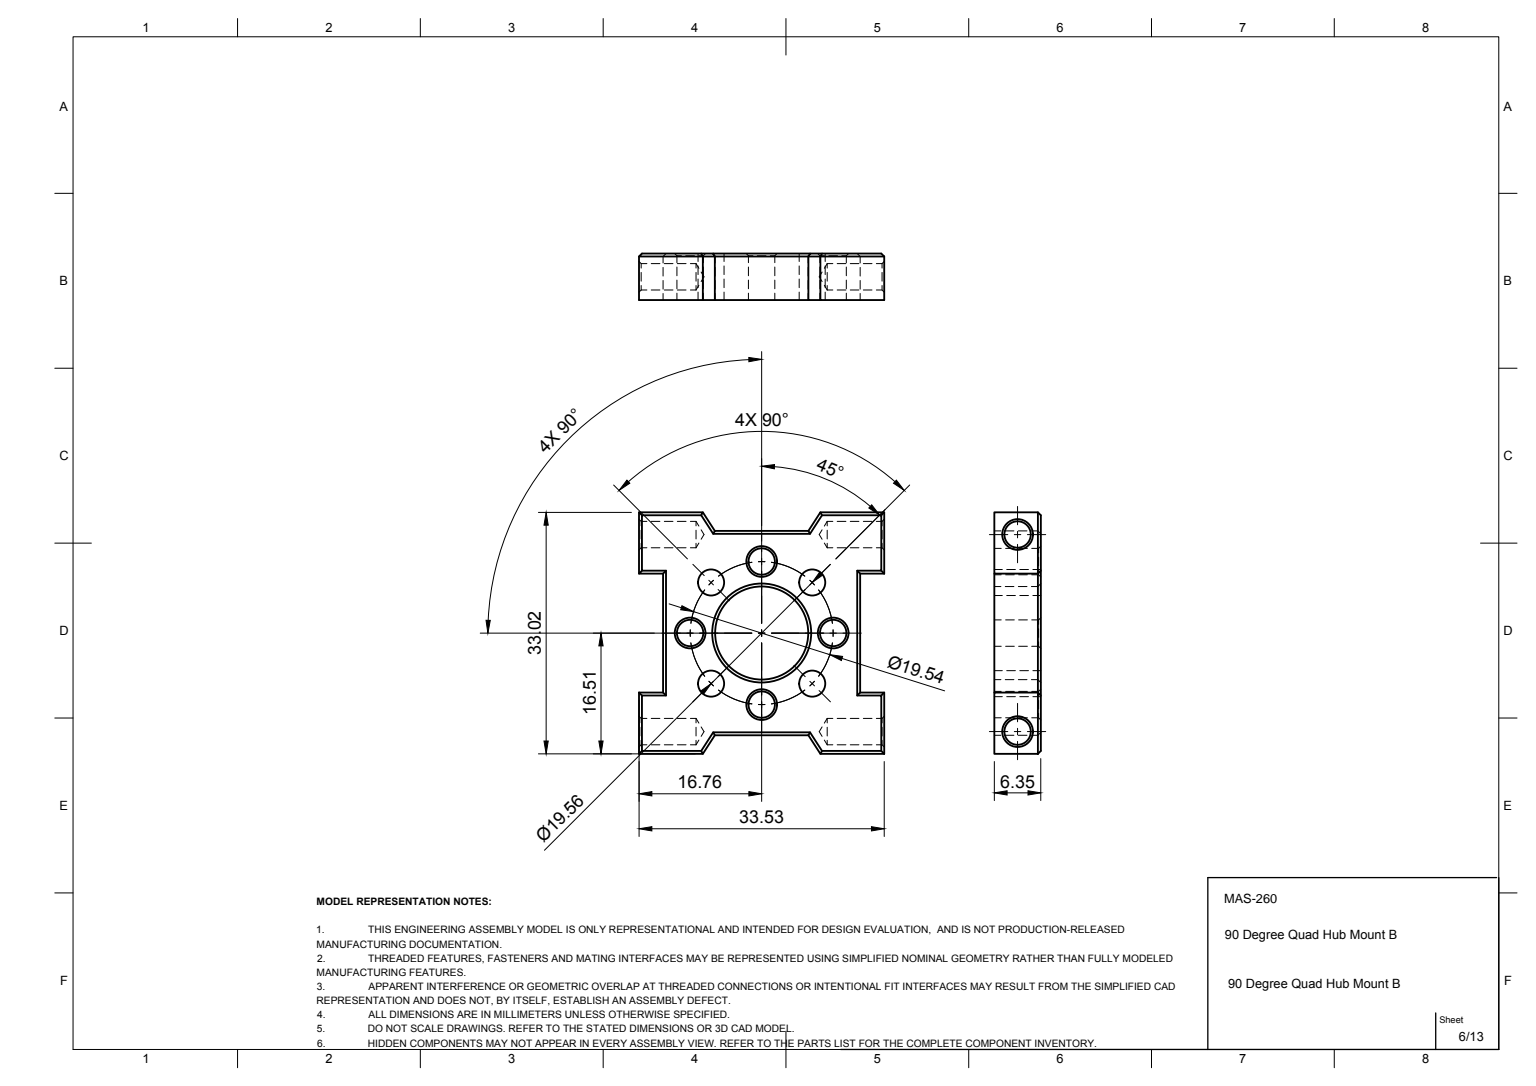
ISO-10303-21;
HEADER;
/* Generated by software containing ST-Developer
 * from STEP Tools, Inc. (www.steptools.com) 
 */

FILE_DESCRIPTION(
/* description */ (''),
/* implementation_level */ '2;1');

FILE_NAME(
/* name */ '90 Degree Quad Hub Mount B.step',
/* time_stamp */ '2026-10-15T13:29:10-07:00',
/* author */ (''),
/* organization */ (''),
/* preprocessor_version */ 'ST-DEVELOPER v20.2',
/* originating_system */ 'Autodesk Translation Framework v15.15.0.0',
/* authorisation */ '');

FILE_SCHEMA (('AUTOMOTIVE_DESIGN { 1 0 10303 214 3 1 1 }'));
ENDSEC;

DATA;
#10=MECHANICAL_DESIGN_GEOMETRIC_PRESENTATION_REPRESENTATION('',(#933),#83219);
#905=SHAPE_REPRESENTATION_RELATIONSHIP('SRR','None',#83300,#919);
#919=ADVANCED_BREP_SHAPE_REPRESENTATION('',(#947),#83205);
#933=STYLED_ITEM('',(#83379),#947);
#947=MANIFOLD_SOLID_BREP('Body1',#26929);
#961=FACE_BOUND('',#3739,.T.);
#962=FACE_BOUND('',#3743,.T.);
#963=FACE_BOUND('',#3749,.T.);
#964=FACE_BOUND('',#3753,.T.);
#965=FACE_BOUND('',#3762,.T.);
#966=FACE_BOUND('',#3763,.T.);
#967=FACE_BOUND('',#3764,.T.);
#968=FACE_BOUND('',#3765,.T.);
#969=FACE_BOUND('',#3766,.T.);
#970=FACE_BOUND('',#3767,.T.);
#971=FACE_BOUND('',#3768,.T.);
#972=FACE_BOUND('',#3769,.T.);
#973=FACE_BOUND('',#3770,.T.);
#974=FACE_BOUND('',#3814,.T.);
#975=FACE_BOUND('',#3815,.T.);
#976=FACE_BOUND('',#3816,.T.);
#977=FACE_BOUND('',#3817,.T.);
#978=FACE_BOUND('',#3818,.T.);
#979=FACE_BOUND('',#3819,.T.);
#980=FACE_BOUND('',#3820,.T.);
#981=FACE_BOUND('',#3821,.T.);
#982=FACE_BOUND('',#3822,.T.);
#1123=PLANE('',#27106);
#1124=PLANE('',#27113);
#1125=PLANE('',#27122);
#1126=PLANE('',#27129);
#1127=PLANE('',#27147);
#1128=PLANE('',#27170);
#1129=PLANE('',#27171);
#1130=PLANE('',#27172);
#1131=PLANE('',#27173);
#1132=PLANE('',#27174);
#1133=PLANE('',#27175);
#1134=PLANE('',#27176);
#1135=PLANE('',#27177);
#1136=PLANE('',#27178);
#1137=PLANE('',#27179);
#1138=PLANE('',#27180);
#1139=PLANE('',#27181);
#1140=PLANE('',#27182);
#1141=PLANE('',#27183);
#1142=PLANE('',#27184);
#1143=PLANE('',#27185);
#1144=PLANE('',#27186);
#1145=PLANE('',#27187);
#1146=PLANE('',#27188);
#1147=PLANE('',#27189);
#1148=PLANE('',#27190);
#1149=PLANE('',#27191);
#1150=PLANE('',#27192);
#1151=PLANE('',#27193);
#1152=PLANE('',#27194);
#1153=PLANE('',#27195);
#1154=PLANE('',#27196);
#1155=PLANE('',#27197);
#1156=PLANE('',#27198);
#1157=PLANE('',#27199);
#1158=PLANE('',#27200);
#1159=PLANE('',#27201);
#1160=PLANE('',#27202);
#1161=PLANE('',#27203);
#1162=PLANE('',#27204);
#1163=PLANE('',#27205);
#1164=PLANE('',#27206);
#2142=CYLINDRICAL_SURFACE('',#27103,1.8025);
#2143=CYLINDRICAL_SURFACE('',#27110,1.8025);
#2144=CYLINDRICAL_SURFACE('',#27119,1.8025);
#2145=CYLINDRICAL_SURFACE('',#27126,1.8025);
#2146=CYLINDRICAL_SURFACE('',#27132,1.778);
#2147=CYLINDRICAL_SURFACE('',#27135,1.778);
#2148=CYLINDRICAL_SURFACE('',#27138,1.778);
#2149=CYLINDRICAL_SURFACE('',#27141,1.778);
#2150=CYLINDRICAL_SURFACE('',#27152,1.8025);
#2151=CYLINDRICAL_SURFACE('',#27156,1.8025);
#2152=CYLINDRICAL_SURFACE('',#27160,1.8025);
#2153=CYLINDRICAL_SURFACE('',#27164,1.8025);
#2154=CYLINDRICAL_SURFACE('',#27168,6.363);
#2357=FACE_OUTER_BOUND('',#3736,.T.);
#2358=FACE_OUTER_BOUND('',#3737,.T.);
#2359=FACE_OUTER_BOUND('',#3738,.T.);
#2360=FACE_OUTER_BOUND('',#3740,.T.);
#2361=FACE_OUTER_BOUND('',#3741,.T.);
#2362=FACE_OUTER_BOUND('',#3742,.T.);
#2363=FACE_OUTER_BOUND('',#3744,.T.);
#2364=FACE_OUTER_BOUND('',#3745,.T.);
#2365=FACE_OUTER_BOUND('',#3746,.T.);
#2366=FACE_OUTER_BOUND('',#3747,.T.);
#2367=FACE_OUTER_BOUND('',#3748,.T.);
#2368=FACE_OUTER_BOUND('',#3750,.T.);
#2369=FACE_OUTER_BOUND('',#3751,.T.);
#2370=FACE_OUTER_BOUND('',#3752,.T.);
#2371=FACE_OUTER_BOUND('',#3754,.T.);
#2372=FACE_OUTER_BOUND('',#3755,.T.);
#2373=FACE_OUTER_BOUND('',#3756,.T.);
#2374=FACE_OUTER_BOUND('',#3757,.T.);
#2375=FACE_OUTER_BOUND('',#3758,.T.);
#2376=FACE_OUTER_BOUND('',#3759,.T.);
#2377=FACE_OUTER_BOUND('',#3760,.T.);
#2378=FACE_OUTER_BOUND('',#3761,.T.);
#2379=FACE_OUTER_BOUND('',#3771,.T.);
#2380=FACE_OUTER_BOUND('',#3772,.T.);
#2381=FACE_OUTER_BOUND('',#3773,.T.);
#2382=FACE_OUTER_BOUND('',#3774,.T.);
#2383=FACE_OUTER_BOUND('',#3775,.T.);
#2384=FACE_OUTER_BOUND('',#3776,.T.);
#2385=FACE_OUTER_BOUND('',#3777,.T.);
#2386=FACE_OUTER_BOUND('',#3778,.T.);
#2387=FACE_OUTER_BOUND('',#3779,.T.);
#2388=FACE_OUTER_BOUND('',#3780,.T.);
#2389=FACE_OUTER_BOUND('',#3781,.T.);
#2390=FACE_OUTER_BOUND('',#3782,.T.);
#2391=FACE_OUTER_BOUND('',#3783,.T.);
#2392=FACE_OUTER_BOUND('',#3784,.T.);
#2393=FACE_OUTER_BOUND('',#3785,.T.);
#2394=FACE_OUTER_BOUND('',#3786,.T.);
#2395=FACE_OUTER_BOUND('',#3787,.T.);
#2396=FACE_OUTER_BOUND('',#3788,.T.);
#2397=FACE_OUTER_BOUND('',#3789,.T.);
#2398=FACE_OUTER_BOUND('',#3790,.T.);
#2399=FACE_OUTER_BOUND('',#3791,.T.);
#2400=FACE_OUTER_BOUND('',#3792,.T.);
#2401=FACE_OUTER_BOUND('',#3793,.T.);
#2402=FACE_OUTER_BOUND('',#3794,.T.);
#2403=FACE_OUTER_BOUND('',#3795,.T.);
#2404=FACE_OUTER_BOUND('',#3796,.T.);
#2405=FACE_OUTER_BOUND('',#3797,.T.);
#2406=FACE_OUTER_BOUND('',#3798,.T.);
#2407=FACE_OUTER_BOUND('',#3799,.T.);
#2408=FACE_OUTER_BOUND('',#3800,.T.);
#2409=FACE_OUTER_BOUND('',#3801,.T.);
#2410=FACE_OUTER_BOUND('',#3802,.T.);
#2411=FACE_OUTER_BOUND('',#3803,.T.);
#2412=FACE_OUTER_BOUND('',#3804,.T.);
#2413=FACE_OUTER_BOUND('',#3805,.T.);
#2414=FACE_OUTER_BOUND('',#3806,.T.);
#2415=FACE_OUTER_BOUND('',#3807,.T.);
#2416=FACE_OUTER_BOUND('',#3808,.T.);
#2417=FACE_OUTER_BOUND('',#3809,.T.);
#2418=FACE_OUTER_BOUND('',#3810,.T.);
#2419=FACE_OUTER_BOUND('',#3811,.T.);
#2420=FACE_OUTER_BOUND('',#3812,.T.);
#2421=FACE_OUTER_BOUND('',#3813,.T.);
#2422=FACE_OUTER_BOUND('',#3823,.T.);
#2423=FACE_OUTER_BOUND('',#3824,.T.);
#2424=FACE_OUTER_BOUND('',#3825,.T.);
#3736=EDGE_LOOP('',(#17586,#17587,#17588,#17589));
#3737=EDGE_LOOP('',(#17590,#17591,#17592,#17593,#17594));
#3738=EDGE_LOOP('',(#17595,#17596,#17597,#17598));
#3739=EDGE_LOOP('',(#17599));
#3740=EDGE_LOOP('',(#17600,#17601,#17602,#17603));
#3741=EDGE_LOOP('',(#17604,#17605,#17606,#17607,#17608));
#3742=EDGE_LOOP('',(#17609,#17610,#17611,#17612));
#3743=EDGE_LOOP('',(#17613));
#3744=EDGE_LOOP('',(#17614,#17615,#17616,#17617));
#3745=EDGE_LOOP('',(#17618,#17619,#17620,#17621));
#3746=EDGE_LOOP('',(#17622,#17623,#17624,#17625));
#3747=EDGE_LOOP('',(#17626,#17627,#17628,#17629,#17630));
#3748=EDGE_LOOP('',(#17631,#17632,#17633,#17634));
#3749=EDGE_LOOP('',(#17635));
#3750=EDGE_LOOP('',(#17636,#17637,#17638,#17639));
#3751=EDGE_LOOP('',(#17640,#17641,#17642,#17643,#17644));
#3752=EDGE_LOOP('',(#17645,#17646,#17647,#17648));
#3753=EDGE_LOOP('',(#17649));
#3754=EDGE_LOOP('',(#17650,#17651,#17652,#17653));
#3755=EDGE_LOOP('',(#17654,#17655,#17656,#17657));
#3756=EDGE_LOOP('',(#17658,#17659,#17660,#17661));
#3757=EDGE_LOOP('',(#17662,#17663,#17664,#17665));
#3758=EDGE_LOOP('',(#17666,#17667,#17668,#17669));
#3759=EDGE_LOOP('',(#17670,#17671,#17672,#17673));
#3760=EDGE_LOOP('',(#17674,#17675,#17676,#17677));
#3761=EDGE_LOOP('',(#17678,#17679,#17680,#17681,#17682,#17683,#17684,#17685,
#17686,#17687,#17688,#17689,#17690,#17691,#17692,#17693,#17694,#17695,#17696,
#17697));
#3762=EDGE_LOOP('',(#17698));
#3763=EDGE_LOOP('',(#17699));
#3764=EDGE_LOOP('',(#17700));
#3765=EDGE_LOOP('',(#17701));
#3766=EDGE_LOOP('',(#17702));
#3767=EDGE_LOOP('',(#17703));
#3768=EDGE_LOOP('',(#17704));
#3769=EDGE_LOOP('',(#17705));
#3770=EDGE_LOOP('',(#17706));
#3771=EDGE_LOOP('',(#17707,#17708,#17709,#17710));
#3772=EDGE_LOOP('',(#17711,#17712,#17713,#17714));
#3773=EDGE_LOOP('',(#17715,#17716,#17717,#17718));
#3774=EDGE_LOOP('',(#17719,#17720,#17721,#17722));
#3775=EDGE_LOOP('',(#17723,#17724,#17725,#17726));
#3776=EDGE_LOOP('',(#17727,#17728,#17729,#17730));
#3777=EDGE_LOOP('',(#17731,#17732,#17733,#17734));
#3778=EDGE_LOOP('',(#17735,#17736,#17737,#17738));
#3779=EDGE_LOOP('',(#17739,#17740,#17741,#17742));
#3780=EDGE_LOOP('',(#17743,#17744,#17745,#17746));
#3781=EDGE_LOOP('',(#17747,#17748,#17749,#17750));
#3782=EDGE_LOOP('',(#17751,#17752,#17753,#17754));
#3783=EDGE_LOOP('',(#17755,#17756,#17757,#17758));
#3784=EDGE_LOOP('',(#17759,#17760,#17761,#17762));
#3785=EDGE_LOOP('',(#17763,#17764,#17765,#17766));
#3786=EDGE_LOOP('',(#17767,#17768,#17769,#17770));
#3787=EDGE_LOOP('',(#17771,#17772,#17773,#17774));
#3788=EDGE_LOOP('',(#17775,#17776,#17777,#17778));
#3789=EDGE_LOOP('',(#17779,#17780,#17781,#17782));
#3790=EDGE_LOOP('',(#17783,#17784,#17785,#17786));
#3791=EDGE_LOOP('',(#17787,#17788,#17789,#17790));
#3792=EDGE_LOOP('',(#17791,#17792,#17793,#17794));
#3793=EDGE_LOOP('',(#17795,#17796,#17797,#17798));
#3794=EDGE_LOOP('',(#17799,#17800,#17801,#17802));
#3795=EDGE_LOOP('',(#17803,#17804,#17805,#17806));
#3796=EDGE_LOOP('',(#17807,#17808,#17809,#17810));
#3797=EDGE_LOOP('',(#17811,#17812,#17813,#17814));
#3798=EDGE_LOOP('',(#17815,#17816,#17817,#17818));
#3799=EDGE_LOOP('',(#17819,#17820,#17821,#17822));
#3800=EDGE_LOOP('',(#17823,#17824,#17825,#17826));
#3801=EDGE_LOOP('',(#17827,#17828,#17829,#17830));
#3802=EDGE_LOOP('',(#17831,#17832,#17833,#17834));
#3803=EDGE_LOOP('',(#17835,#17836,#17837,#17838));
#3804=EDGE_LOOP('',(#17839,#17840,#17841,#17842));
#3805=EDGE_LOOP('',(#17843,#17844,#17845,#17846));
#3806=EDGE_LOOP('',(#17847,#17848,#17849,#17850));
#3807=EDGE_LOOP('',(#17851,#17852,#17853,#17854));
#3808=EDGE_LOOP('',(#17855,#17856,#17857,#17858));
#3809=EDGE_LOOP('',(#17859,#17860,#17861,#17862));
#3810=EDGE_LOOP('',(#17863,#17864,#17865,#17866));
#3811=EDGE_LOOP('',(#17867,#17868,#17869,#17870));
#3812=EDGE_LOOP('',(#17871,#17872,#17873,#17874));
#3813=EDGE_LOOP('',(#17875,#17876,#17877,#17878,#17879,#17880,#17881,#17882,
#17883,#17884,#17885,#17886,#17887,#17888,#17889,#17890,#17891,#17892,#17893,
#17894));
#3814=EDGE_LOOP('',(#17895));
#3815=EDGE_LOOP('',(#17896));
#3816=EDGE_LOOP('',(#17897));
#3817=EDGE_LOOP('',(#17898));
#3818=EDGE_LOOP('',(#17899));
#3819=EDGE_LOOP('',(#17900));
#3820=EDGE_LOOP('',(#17901));
#3821=EDGE_LOOP('',(#17902));
#3822=EDGE_LOOP('',(#17903));
#3823=EDGE_LOOP('',(#17904,#17905,#17906,#17907));
#3824=EDGE_LOOP('',(#17908,#17909,#17910,#17911));
#3825=EDGE_LOOP('',(#17912,#17913,#17914,#17915));
#5277=LINE('',#36086,#7788);
#5278=LINE('',#36090,#7789);
#5279=LINE('',#36097,#7790);
#5280=LINE('',#36099,#7791);
#5281=LINE('',#36101,#7792);
#5282=LINE('',#36102,#7793);
#5283=LINE('',#36107,#7794);
#5284=LINE('',#36111,#7795);
#5285=LINE('',#36118,#7796);
#5286=LINE('',#36120,#7797);
#5287=LINE('',#36122,#7798);
#5288=LINE('',#36123,#7799);
#5289=LINE('',#36126,#7800);
#5290=LINE('',#36129,#7801);
#5291=LINE('',#36134,#7802);
#5292=LINE('',#36138,#7803);
#5293=LINE('',#36145,#7804);
#5294=LINE('',#36147,#7805);
#5295=LINE('',#36149,#7806);
#5296=LINE('',#36150,#7807);
#5297=LINE('',#36155,#7808);
#5298=LINE('',#36159,#7809);
#5299=LINE('',#36166,#7810);
#5300=LINE('',#36168,#7811);
#5301=LINE('',#36170,#7812);
#5302=LINE('',#36171,#7813);
#5303=LINE('',#36174,#7814);
#5304=LINE('',#36177,#7815);
#5305=LINE('',#36182,#7816);
#5306=LINE('',#36188,#7817);
#5307=LINE('',#36194,#7818);
#5308=LINE('',#36200,#7819);
#5309=LINE('',#36206,#7820);
#5310=LINE('',#36211,#7821);
#5311=LINE('',#36213,#7822);
#5312=LINE('',#36215,#7823);
#5313=LINE('',#36217,#7824);
#5314=LINE('',#36219,#7825);
#5315=LINE('',#36221,#7826);
#5316=LINE('',#36223,#7827);
#5317=LINE('',#36225,#7828);
#5318=LINE('',#36227,#7829);
#5319=LINE('',#36229,#7830);
#5320=LINE('',#36231,#7831);
#5321=LINE('',#36233,#7832);
#5322=LINE('',#36235,#7833);
#5323=LINE('',#36237,#7834);
#5324=LINE('',#36239,#7835);
#5325=LINE('',#36241,#7836);
#5326=LINE('',#36243,#7837);
#5327=LINE('',#36245,#7838);
#5328=LINE('',#36247,#7839);
#5329=LINE('',#36248,#7840);
#5330=LINE('',#36259,#7841);
#5331=LINE('',#36264,#7842);
#5332=LINE('',#36267,#7843);
#5333=LINE('',#36272,#7844);
#5334=LINE('',#36275,#7845);
#5335=LINE('',#36280,#7846);
#5336=LINE('',#36283,#7847);
#5337=LINE('',#36288,#7848);
#5338=LINE('',#36291,#7849);
#5339=LINE('',#36295,#7850);
#5340=LINE('',#36297,#7851);
#5341=LINE('',#36298,#7852);
#5342=LINE('',#36300,#7853);
#5343=LINE('',#36301,#7854);
#5344=LINE('',#36303,#7855);
#5345=LINE('',#36307,#7856);
#5346=LINE('',#36308,#7857);
#5347=LINE('',#36309,#7858);
#5348=LINE('',#36312,#7859);
#5349=LINE('',#36313,#7860);
#5350=LINE('',#36315,#7861);
#5351=LINE('',#36317,#7862);
#5352=LINE('',#36318,#7863);
#5353=LINE('',#36320,#7864);
#5354=LINE('',#36324,#7865);
#5355=LINE('',#36325,#7866);
#5356=LINE('',#36326,#7867);
#5357=LINE('',#36329,#7868);
#5358=LINE('',#36330,#7869);
#5359=LINE('',#36333,#7870);
#5360=LINE('',#36334,#7871);
#5361=LINE('',#36336,#7872);
#5362=LINE('',#36338,#7873);
#5363=LINE('',#36339,#7874);
#5364=LINE('',#36341,#7875);
#5365=LINE('',#36343,#7876);
#5366=LINE('',#36345,#7877);
#5367=LINE('',#36347,#7878);
#5368=LINE('',#36348,#7879);
#5369=LINE('',#36350,#7880);
#5370=LINE('',#36353,#7881);
#5371=LINE('',#36354,#7882);
#5372=LINE('',#36357,#7883);
#5373=LINE('',#36358,#7884);
#5374=LINE('',#36360,#7885);
#5375=LINE('',#36363,#7886);
#5376=LINE('',#36364,#7887);
#5377=LINE('',#36367,#7888);
#5378=LINE('',#36368,#7889);
#5379=LINE('',#36371,#7890);
#5380=LINE('',#36372,#7891);
#5381=LINE('',#36374,#7892);
#5382=LINE('',#36377,#7893);
#5383=LINE('',#36378,#7894);
#5384=LINE('',#36381,#7895);
#5385=LINE('',#36382,#7896);
#5386=LINE('',#36385,#7897);
#5387=LINE('',#36386,#7898);
#5388=LINE('',#36389,#7899);
#5389=LINE('',#36390,#7900);
#5390=LINE('',#36393,#7901);
#5391=LINE('',#36395,#7902);
#5392=LINE('',#36396,#7903);
#5393=LINE('',#36399,#7904);
#5394=LINE('',#36400,#7905);
#5395=LINE('',#36402,#7906);
#5396=LINE('',#36404,#7907);
#5397=LINE('',#36406,#7908);
#5398=LINE('',#36409,#7909);
#5399=LINE('',#36411,#7910);
#5400=LINE('',#36412,#7911);
#5401=LINE('',#36414,#7912);
#5402=LINE('',#36415,#7913);
#7788=VECTOR('',#29263,1.9525);
#7789=VECTOR('',#29268,1.8025);
#7790=VECTOR('',#29275,10.);
#7791=VECTOR('',#29276,10.);
#7792=VECTOR('',#29277,10.);
#7793=VECTOR('',#29278,10.);
#7794=VECTOR('',#29283,1.9525);
#7795=VECTOR('',#29288,1.8025);
#7796=VECTOR('',#29295,10.);
#7797=VECTOR('',#29296,10.);
#7798=VECTOR('',#29297,10.);
#7799=VECTOR('',#29298,10.);
#7800=VECTOR('',#29301,1.80249999999999);
#7801=VECTOR('',#29304,1.80249999999999);
#7802=VECTOR('',#29309,1.9525);
#7803=VECTOR('',#29314,1.8025);
#7804=VECTOR('',#29321,10.);
#7805=VECTOR('',#29322,10.);
#7806=VECTOR('',#29323,10.);
#7807=VECTOR('',#29324,10.);
#7808=VECTOR('',#29329,1.9525);
#7809=VECTOR('',#29334,1.8025);
#7810=VECTOR('',#29341,10.);
#7811=VECTOR('',#29342,10.);
#7812=VECTOR('',#29343,10.);
#7813=VECTOR('',#29344,10.);
#7814=VECTOR('',#29347,0.901249999999996);
#7815=VECTOR('',#29350,0.901249999999996);
#7816=VECTOR('',#29355,1.778);
#7817=VECTOR('',#29362,1.778);
#7818=VECTOR('',#29369,1.778);
#7819=VECTOR('',#29376,1.778);
#7820=VECTOR('',#29383,1.9525);
#7821=VECTOR('',#29388,10.);
#7822=VECTOR('',#29389,10.);
#7823=VECTOR('',#29390,10.);
#7824=VECTOR('',#29391,10.);
#7825=VECTOR('',#29392,10.);
#7826=VECTOR('',#29393,10.);
#7827=VECTOR('',#29394,10.);
#7828=VECTOR('',#29395,10.);
#7829=VECTOR('',#29396,10.);
#7830=VECTOR('',#29397,10.);
#7831=VECTOR('',#29398,10.);
#7832=VECTOR('',#29399,10.);
#7833=VECTOR('',#29400,10.);
#7834=VECTOR('',#29401,10.);
#7835=VECTOR('',#29402,10.);
#7836=VECTOR('',#29403,10.);
#7837=VECTOR('',#29404,10.);
#7838=VECTOR('',#29405,10.);
#7839=VECTOR('',#29406,10.);
#7840=VECTOR('',#29407,10.);
#7841=VECTOR('',#29418,1.8025);
#7842=VECTOR('',#29425,1.9525);
#7843=VECTOR('',#29428,1.8025);
#7844=VECTOR('',#29435,1.9525);
#7845=VECTOR('',#29438,1.8025);
#7846=VECTOR('',#29445,1.9525);
#7847=VECTOR('',#29448,1.8025);
#7848=VECTOR('',#29455,6.563);
#7849=VECTOR('',#29458,6.363);
#7850=VECTOR('',#29463,10.);
#7851=VECTOR('',#29464,10.);
#7852=VECTOR('',#29465,10.);
#7853=VECTOR('',#29468,9.99999999999999);
#7854=VECTOR('',#29469,10.);
#7855=VECTOR('',#29472,10.);
#7856=VECTOR('',#29475,10.);
#7857=VECTOR('',#29476,10.);
#7858=VECTOR('',#29477,10.);
#7859=VECTOR('',#29480,10.);
#7860=VECTOR('',#29481,10.);
#7861=VECTOR('',#29484,10.);
#7862=VECTOR('',#29485,10.);
#7863=VECTOR('',#29486,10.);
#7864=VECTOR('',#29489,10.);
#7865=VECTOR('',#29492,10.);
#7866=VECTOR('',#29493,10.);
#7867=VECTOR('',#29494,10.);
#7868=VECTOR('',#29497,10.);
#7869=VECTOR('',#29498,10.);
#7870=VECTOR('',#29501,10.);
#7871=VECTOR('',#29502,10.);
#7872=VECTOR('',#29505,10.);
#7873=VECTOR('',#29508,10.);
#7874=VECTOR('',#29509,9.99999999999999);
#7875=VECTOR('',#29512,10.);
#7876=VECTOR('',#29515,10.);
#7877=VECTOR('',#29518,10.);
#7878=VECTOR('',#29521,10.);
#7879=VECTOR('',#29522,10.);
#7880=VECTOR('',#29525,10.);
#7881=VECTOR('',#29528,10.);
#7882=VECTOR('',#29529,10.);
#7883=VECTOR('',#29532,10.);
#7884=VECTOR('',#29533,10.);
#7885=VECTOR('',#29536,10.);
#7886=VECTOR('',#29539,10.);
#7887=VECTOR('',#29540,10.);
#7888=VECTOR('',#29543,10.);
#7889=VECTOR('',#29544,10.);
#7890=VECTOR('',#29547,10.);
#7891=VECTOR('',#29548,10.);
#7892=VECTOR('',#29551,10.);
#7893=VECTOR('',#29554,10.);
#7894=VECTOR('',#29555,10.);
#7895=VECTOR('',#29558,10.);
#7896=VECTOR('',#29559,10.);
#7897=VECTOR('',#29562,10.);
#7898=VECTOR('',#29563,10.);
#7899=VECTOR('',#29566,10.);
#7900=VECTOR('',#29567,10.);
#7901=VECTOR('',#29570,10.);
#7902=VECTOR('',#29571,10.);
#7903=VECTOR('',#29572,10.);
#7904=VECTOR('',#29575,10.);
#7905=VECTOR('',#29576,10.);
#7906=VECTOR('',#29579,10.);
#7907=VECTOR('',#29582,10.);
#7908=VECTOR('',#29585,10.);
#7909=VECTOR('',#29588,10.);
#7910=VECTOR('',#29589,10.);
#7911=VECTOR('',#29590,10.);
#7912=VECTOR('',#29593,10.);
#7913=VECTOR('',#29594,10.);
#10299=CIRCLE('',#27101,1.8025);
#10300=CIRCLE('',#27102,2.1025);
#10301=CIRCLE('',#27104,1.8025);
#10302=CIRCLE('',#27105,1.8025);
#10303=CIRCLE('',#27108,1.8025);
#10304=CIRCLE('',#27109,2.1025);
#10305=CIRCLE('',#27111,1.8025);
#10306=CIRCLE('',#27112,1.8025);
#10307=CIRCLE('',#27117,1.8025);
#10308=CIRCLE('',#27118,2.1025);
#10309=CIRCLE('',#27120,1.8025);
#10310=CIRCLE('',#27121,1.8025);
#10311=CIRCLE('',#27124,1.8025);
#10312=CIRCLE('',#27125,2.1025);
#10313=CIRCLE('',#27127,1.8025);
#10314=CIRCLE('',#27128,1.8025);
#10315=CIRCLE('',#27133,1.778);
#10316=CIRCLE('',#27134,1.778);
#10317=CIRCLE('',#27136,1.778);
#10318=CIRCLE('',#27137,1.778);
#10319=CIRCLE('',#27139,1.778);
#10320=CIRCLE('',#27140,1.778);
#10321=CIRCLE('',#27142,1.778);
#10322=CIRCLE('',#27143,1.778);
#10323=CIRCLE('',#27145,1.8025);
#10324=CIRCLE('',#27146,2.1025);
#10325=CIRCLE('',#27148,2.1025);
#10326=CIRCLE('',#27149,6.763);
#10327=CIRCLE('',#27150,2.1025);
#10328=CIRCLE('',#27151,2.1025);
#10329=CIRCLE('',#27153,1.8025);
#10330=CIRCLE('',#27155,1.8025);
#10331=CIRCLE('',#27157,1.8025);
#10332=CIRCLE('',#27159,1.8025);
#10333=CIRCLE('',#27161,1.8025);
#10334=CIRCLE('',#27163,1.8025);
#10335=CIRCLE('',#27165,1.8025);
#10336=CIRCLE('',#27167,6.363);
#10337=CIRCLE('',#27169,6.363);
#11051=VERTEX_POINT('',#36083);
#11052=VERTEX_POINT('',#36085);
#11053=VERTEX_POINT('',#36089);
#11054=VERTEX_POINT('',#36091);
#11055=VERTEX_POINT('',#36095);
#11056=VERTEX_POINT('',#36096);
#11057=VERTEX_POINT('',#36098);
#11058=VERTEX_POINT('',#36100);
#11059=VERTEX_POINT('',#36104);
#11060=VERTEX_POINT('',#36106);
#11061=VERTEX_POINT('',#36110);
#11062=VERTEX_POINT('',#36112);
#11063=VERTEX_POINT('',#36116);
#11064=VERTEX_POINT('',#36117);
#11065=VERTEX_POINT('',#36119);
#11066=VERTEX_POINT('',#36121);
#11067=VERTEX_POINT('',#36125);
#11068=VERTEX_POINT('',#36128);
#11069=VERTEX_POINT('',#36131);
#11070=VERTEX_POINT('',#36133);
#11071=VERTEX_POINT('',#36137);
#11072=VERTEX_POINT('',#36139);
#11073=VERTEX_POINT('',#36143);
#11074=VERTEX_POINT('',#36144);
#11075=VERTEX_POINT('',#36146);
#11076=VERTEX_POINT('',#36148);
#11077=VERTEX_POINT('',#36152);
#11078=VERTEX_POINT('',#36154);
#11079=VERTEX_POINT('',#36158);
#11080=VERTEX_POINT('',#36160);
#11081=VERTEX_POINT('',#36164);
#11082=VERTEX_POINT('',#36165);
#11083=VERTEX_POINT('',#36167);
#11084=VERTEX_POINT('',#36169);
#11085=VERTEX_POINT('',#36173);
#11086=VERTEX_POINT('',#36176);
#11087=VERTEX_POINT('',#36179);
#11088=VERTEX_POINT('',#36181);
#11089=VERTEX_POINT('',#36185);
#11090=VERTEX_POINT('',#36187);
#11091=VERTEX_POINT('',#36191);
#11092=VERTEX_POINT('',#36193);
#11093=VERTEX_POINT('',#36197);
#11094=VERTEX_POINT('',#36199);
#11095=VERTEX_POINT('',#36203);
#11096=VERTEX_POINT('',#36205);
#11097=VERTEX_POINT('',#36209);
#11098=VERTEX_POINT('',#36210);
#11099=VERTEX_POINT('',#36212);
#11100=VERTEX_POINT('',#36214);
#11101=VERTEX_POINT('',#36216);
#11102=VERTEX_POINT('',#36218);
#11103=VERTEX_POINT('',#36220);
#11104=VERTEX_POINT('',#36222);
#11105=VERTEX_POINT('',#36224);
#11106=VERTEX_POINT('',#36226);
#11107=VERTEX_POINT('',#36228);
#11108=VERTEX_POINT('',#36230);
#11109=VERTEX_POINT('',#36232);
#11110=VERTEX_POINT('',#36234);
#11111=VERTEX_POINT('',#36236);
#11112=VERTEX_POINT('',#36238);
#11113=VERTEX_POINT('',#36240);
#11114=VERTEX_POINT('',#36242);
#11115=VERTEX_POINT('',#36244);
#11116=VERTEX_POINT('',#36246);
#11117=VERTEX_POINT('',#36249);
#11118=VERTEX_POINT('',#36251);
#11119=VERTEX_POINT('',#36253);
#11120=VERTEX_POINT('',#36255);
#11121=VERTEX_POINT('',#36258);
#11122=VERTEX_POINT('',#36262);
#11123=VERTEX_POINT('',#36266);
#11124=VERTEX_POINT('',#36270);
#11125=VERTEX_POINT('',#36274);
#11126=VERTEX_POINT('',#36278);
#11127=VERTEX_POINT('',#36282);
#11128=VERTEX_POINT('',#36286);
#11129=VERTEX_POINT('',#36290);
#11130=VERTEX_POINT('',#36294);
#11131=VERTEX_POINT('',#36296);
#11132=VERTEX_POINT('',#36305);
#11133=VERTEX_POINT('',#36306);
#11134=VERTEX_POINT('',#36311);
#11135=VERTEX_POINT('',#36316);
#11136=VERTEX_POINT('',#36322);
#11137=VERTEX_POINT('',#36323);
#11138=VERTEX_POINT('',#36328);
#11139=VERTEX_POINT('',#36332);
#11140=VERTEX_POINT('',#36352);
#11141=VERTEX_POINT('',#36356);
#11142=VERTEX_POINT('',#36362);
#11143=VERTEX_POINT('',#36366);
#11144=VERTEX_POINT('',#36370);
#11145=VERTEX_POINT('',#36376);
#11146=VERTEX_POINT('',#36380);
#11147=VERTEX_POINT('',#36384);
#11148=VERTEX_POINT('',#36388);
#11149=VERTEX_POINT('',#36392);
#11150=VERTEX_POINT('',#36394);
#11151=VERTEX_POINT('',#36398);
#11152=VERTEX_POINT('',#36408);
#11153=VERTEX_POINT('',#36410);
#13654=EDGE_CURVE('',#11051,#11051,#10299,.T.);
#13655=EDGE_CURVE('',#11051,#11052,#5277,.T.);
#13656=EDGE_CURVE('',#11052,#11052,#10300,.T.);
#13657=EDGE_CURVE('',#11051,#11053,#5278,.T.);
#13658=EDGE_CURVE('',#11053,#11054,#10301,.T.);
#13659=EDGE_CURVE('',#11054,#11053,#10302,.T.);
#13660=EDGE_CURVE('',#11055,#11056,#5279,.T.);
#13661=EDGE_CURVE('',#11057,#11055,#5280,.T.);
#13662=EDGE_CURVE('',#11058,#11057,#5281,.T.);
#13663=EDGE_CURVE('',#11058,#11056,#5282,.T.);
#13664=EDGE_CURVE('',#11059,#11059,#10303,.T.);
#13665=EDGE_CURVE('',#11059,#11060,#5283,.T.);
#13666=EDGE_CURVE('',#11060,#11060,#10304,.T.);
#13667=EDGE_CURVE('',#11059,#11061,#5284,.T.);
#13668=EDGE_CURVE('',#11061,#11062,#10305,.T.);
#13669=EDGE_CURVE('',#11062,#11061,#10306,.T.);
#13670=EDGE_CURVE('',#11063,#11064,#5285,.T.);
#13671=EDGE_CURVE('',#11063,#11065,#5286,.T.);
#13672=EDGE_CURVE('',#11066,#11065,#5287,.T.);
#13673=EDGE_CURVE('',#11066,#11064,#5288,.T.);
#13674=EDGE_CURVE('',#11067,#11054,#5289,.T.);
#13675=EDGE_CURVE('',#11068,#11062,#5290,.T.);
#13676=EDGE_CURVE('',#11069,#11069,#10307,.T.);
#13677=EDGE_CURVE('',#11069,#11070,#5291,.T.);
#13678=EDGE_CURVE('',#11070,#11070,#10308,.T.);
#13679=EDGE_CURVE('',#11069,#11071,#5292,.T.);
#13680=EDGE_CURVE('',#11071,#11072,#10309,.T.);
#13681=EDGE_CURVE('',#11072,#11071,#10310,.T.);
#13682=EDGE_CURVE('',#11073,#11074,#5293,.T.);
#13683=EDGE_CURVE('',#11073,#11075,#5294,.T.);
#13684=EDGE_CURVE('',#11076,#11075,#5295,.T.);
#13685=EDGE_CURVE('',#11076,#11074,#5296,.T.);
#13686=EDGE_CURVE('',#11077,#11077,#10311,.T.);
#13687=EDGE_CURVE('',#11077,#11078,#5297,.T.);
#13688=EDGE_CURVE('',#11078,#11078,#10312,.T.);
#13689=EDGE_CURVE('',#11077,#11079,#5298,.T.);
#13690=EDGE_CURVE('',#11079,#11080,#10313,.T.);
#13691=EDGE_CURVE('',#11080,#11079,#10314,.T.);
#13692=EDGE_CURVE('',#11081,#11082,#5299,.T.);
#13693=EDGE_CURVE('',#11083,#11081,#5300,.T.);
#13694=EDGE_CURVE('',#11084,#11083,#5301,.T.);
#13695=EDGE_CURVE('',#11084,#11082,#5302,.T.);
#13696=EDGE_CURVE('',#11085,#11072,#5303,.T.);
#13697=EDGE_CURVE('',#11086,#11080,#5304,.T.);
#13698=EDGE_CURVE('',#11087,#11087,#10315,.T.);
#13699=EDGE_CURVE('',#11087,#11088,#5305,.T.);
#13700=EDGE_CURVE('',#11088,#11088,#10316,.T.);
#13701=EDGE_CURVE('',#11089,#11089,#10317,.T.);
#13702=EDGE_CURVE('',#11089,#11090,#5306,.T.);
#13703=EDGE_CURVE('',#11090,#11090,#10318,.T.);
#13704=EDGE_CURVE('',#11091,#11091,#10319,.T.);
#13705=EDGE_CURVE('',#11091,#11092,#5307,.T.);
#13706=EDGE_CURVE('',#11092,#11092,#10320,.T.);
#13707=EDGE_CURVE('',#11093,#11093,#10321,.T.);
#13708=EDGE_CURVE('',#11093,#11094,#5308,.T.);
#13709=EDGE_CURVE('',#11094,#11094,#10322,.T.);
#13710=EDGE_CURVE('',#11095,#11095,#10323,.T.);
#13711=EDGE_CURVE('',#11095,#11096,#5309,.T.);
#13712=EDGE_CURVE('',#11096,#11096,#10324,.T.);
#13713=EDGE_CURVE('',#11097,#11098,#5310,.T.);
#13714=EDGE_CURVE('',#11099,#11097,#5311,.T.);
#13715=EDGE_CURVE('',#11100,#11099,#5312,.T.);
#13716=EDGE_CURVE('',#11101,#11100,#5313,.T.);
#13717=EDGE_CURVE('',#11102,#11101,#5314,.T.);
#13718=EDGE_CURVE('',#11103,#11102,#5315,.T.);
#13719=EDGE_CURVE('',#11104,#11103,#5316,.T.);
#13720=EDGE_CURVE('',#11105,#11104,#5317,.T.);
#13721=EDGE_CURVE('',#11106,#11105,#5318,.T.);
#13722=EDGE_CURVE('',#11107,#11106,#5319,.T.);
#13723=EDGE_CURVE('',#11108,#11107,#5320,.T.);
#13724=EDGE_CURVE('',#11109,#11108,#5321,.T.);
#13725=EDGE_CURVE('',#11110,#11109,#5322,.T.);
#13726=EDGE_CURVE('',#11111,#11110,#5323,.T.);
#13727=EDGE_CURVE('',#11112,#11111,#5324,.T.);
#13728=EDGE_CURVE('',#11113,#11112,#5325,.T.);
#13729=EDGE_CURVE('',#11114,#11113,#5326,.T.);
#13730=EDGE_CURVE('',#11115,#11114,#5327,.T.);
#13731=EDGE_CURVE('',#11116,#11115,#5328,.T.);
#13732=EDGE_CURVE('',#11098,#11116,#5329,.T.);
#13733=EDGE_CURVE('',#11117,#11117,#10325,.T.);
#13734=EDGE_CURVE('',#11118,#11118,#10326,.T.);
#13735=EDGE_CURVE('',#11119,#11119,#10327,.T.);
#13736=EDGE_CURVE('',#11120,#11120,#10328,.T.);
#13737=EDGE_CURVE('',#11095,#11121,#5330,.T.);
#13738=EDGE_CURVE('',#11121,#11121,#10329,.T.);
#13739=EDGE_CURVE('',#11122,#11122,#10330,.T.);
#13740=EDGE_CURVE('',#11122,#11120,#5331,.T.);
#13741=EDGE_CURVE('',#11122,#11123,#5332,.T.);
#13742=EDGE_CURVE('',#11123,#11123,#10331,.T.);
#13743=EDGE_CURVE('',#11124,#11124,#10332,.T.);
#13744=EDGE_CURVE('',#11124,#11117,#5333,.T.);
#13745=EDGE_CURVE('',#11124,#11125,#5334,.T.);
#13746=EDGE_CURVE('',#11125,#11125,#10333,.T.);
#13747=EDGE_CURVE('',#11126,#11126,#10334,.T.);
#13748=EDGE_CURVE('',#11126,#11119,#5335,.T.);
#13749=EDGE_CURVE('',#11126,#11127,#5336,.T.);
#13750=EDGE_CURVE('',#11127,#11127,#10335,.T.);
#13751=EDGE_CURVE('',#11128,#11128,#10336,.T.);
#13752=EDGE_CURVE('',#11128,#11118,#5337,.T.);
#13753=EDGE_CURVE('',#11128,#11129,#5338,.T.);
#13754=EDGE_CURVE('',#11129,#11129,#10337,.T.);
#13755=EDGE_CURVE('',#11107,#11130,#5339,.T.);
#13756=EDGE_CURVE('',#11130,#11131,#5340,.T.);
#13757=EDGE_CURVE('',#11131,#11108,#5341,.T.);
#13758=EDGE_CURVE('',#11106,#11064,#5342,.T.);
#13759=EDGE_CURVE('',#11064,#11130,#5343,.T.);
#13760=EDGE_CURVE('',#11105,#11063,#5344,.T.);
#13761=EDGE_CURVE('',#11132,#11133,#5345,.T.);
#13762=EDGE_CURVE('',#11133,#11114,#5346,.T.);
#13763=EDGE_CURVE('',#11113,#11132,#5347,.T.);
#13764=EDGE_CURVE('',#11104,#11134,#5348,.T.);
#13765=EDGE_CURVE('',#11134,#11063,#5349,.T.);
#13766=EDGE_CURVE('',#11102,#11056,#5350,.T.);
#13767=EDGE_CURVE('',#11056,#11135,#5351,.T.);
#13768=EDGE_CURVE('',#11135,#11103,#5352,.T.);
#13769=EDGE_CURVE('',#11101,#11055,#5353,.T.);
#13770=EDGE_CURVE('',#11136,#11137,#5354,.T.);
#13771=EDGE_CURVE('',#11137,#11097,#5355,.T.);
#13772=EDGE_CURVE('',#11098,#11136,#5356,.T.);
#13773=EDGE_CURVE('',#11100,#11138,#5357,.T.);
#13774=EDGE_CURVE('',#11138,#11055,#5358,.T.);
#13775=EDGE_CURVE('',#11137,#11139,#5359,.T.);
#13776=EDGE_CURVE('',#11139,#11099,#5360,.T.);
#13777=EDGE_CURVE('',#11139,#11138,#5361,.T.);
#13778=EDGE_CURVE('',#11074,#11136,#5362,.T.);
#13779=EDGE_CURVE('',#11116,#11074,#5363,.T.);
#13780=EDGE_CURVE('',#11115,#11073,#5364,.T.);
#13781=EDGE_CURVE('',#11135,#11134,#5365,.T.);
#13782=EDGE_CURVE('',#11133,#11073,#5366,.T.);
#13783=EDGE_CURVE('',#11082,#11132,#5367,.T.);
#13784=EDGE_CURVE('',#11112,#11082,#5368,.T.);
#13785=EDGE_CURVE('',#11111,#11081,#5369,.T.);
#13786=EDGE_CURVE('',#11140,#11081,#5370,.T.);
#13787=EDGE_CURVE('',#11110,#11140,#5371,.T.);
#13788=EDGE_CURVE('',#11131,#11141,#5372,.T.);
#13789=EDGE_CURVE('',#11141,#11109,#5373,.T.);
#13790=EDGE_CURVE('',#11141,#11140,#5374,.T.);
#13791=EDGE_CURVE('',#11142,#11066,#5375,.T.);
#13792=EDGE_CURVE('',#11142,#11130,#5376,.T.);
#13793=EDGE_CURVE('',#11143,#11134,#5377,.T.);
#13794=EDGE_CURVE('',#11065,#11143,#5378,.T.);
#13795=EDGE_CURVE('',#11144,#11135,#5379,.T.);
#13796=EDGE_CURVE('',#11143,#11144,#5380,.T.);
#13797=EDGE_CURVE('',#11144,#11058,#5381,.T.);
#13798=EDGE_CURVE('',#11138,#11145,#5382,.T.);
#13799=EDGE_CURVE('',#11057,#11145,#5383,.T.);
#13800=EDGE_CURVE('',#11146,#11139,#5384,.T.);
#13801=EDGE_CURVE('',#11145,#11146,#5385,.T.);
#13802=EDGE_CURVE('',#11147,#11137,#5386,.T.);
#13803=EDGE_CURVE('',#11146,#11147,#5387,.T.);
#13804=EDGE_CURVE('',#11148,#11136,#5388,.T.);
#13805=EDGE_CURVE('',#11147,#11148,#5389,.T.);
#13806=EDGE_CURVE('',#11149,#11141,#5390,.T.);
#13807=EDGE_CURVE('',#11150,#11149,#5391,.T.);
#13808=EDGE_CURVE('',#11140,#11150,#5392,.T.);
#13809=EDGE_CURVE('',#11151,#11142,#5393,.T.);
#13810=EDGE_CURVE('',#11151,#11131,#5394,.T.);
#13811=EDGE_CURVE('',#11149,#11151,#5395,.T.);
#13812=EDGE_CURVE('',#11148,#11076,#5396,.T.);
#13813=EDGE_CURVE('',#11083,#11150,#5397,.T.);
#13814=EDGE_CURVE('',#11075,#11152,#5398,.T.);
#13815=EDGE_CURVE('',#11152,#11153,#5399,.T.);
#13816=EDGE_CURVE('',#11153,#11084,#5400,.T.);
#13817=EDGE_CURVE('',#11153,#11132,#5401,.T.);
#13818=EDGE_CURVE('',#11152,#11133,#5402,.T.);
#17586=ORIENTED_EDGE('',*,*,#13654,.T.);
#17587=ORIENTED_EDGE('',*,*,#13655,.T.);
#17588=ORIENTED_EDGE('',*,*,#13656,.T.);
#17589=ORIENTED_EDGE('',*,*,#13655,.F.);
#17590=ORIENTED_EDGE('',*,*,#13654,.F.);
#17591=ORIENTED_EDGE('',*,*,#13657,.T.);
#17592=ORIENTED_EDGE('',*,*,#13658,.T.);
#17593=ORIENTED_EDGE('',*,*,#13659,.T.);
#17594=ORIENTED_EDGE('',*,*,#13657,.F.);
#17595=ORIENTED_EDGE('',*,*,#13660,.F.);
#17596=ORIENTED_EDGE('',*,*,#13661,.F.);
#17597=ORIENTED_EDGE('',*,*,#13662,.F.);
#17598=ORIENTED_EDGE('',*,*,#13663,.T.);
#17599=ORIENTED_EDGE('',*,*,#13656,.F.);
#17600=ORIENTED_EDGE('',*,*,#13664,.T.);
#17601=ORIENTED_EDGE('',*,*,#13665,.T.);
#17602=ORIENTED_EDGE('',*,*,#13666,.T.);
#17603=ORIENTED_EDGE('',*,*,#13665,.F.);
#17604=ORIENTED_EDGE('',*,*,#13664,.F.);
#17605=ORIENTED_EDGE('',*,*,#13667,.T.);
#17606=ORIENTED_EDGE('',*,*,#13668,.T.);
#17607=ORIENTED_EDGE('',*,*,#13669,.T.);
#17608=ORIENTED_EDGE('',*,*,#13667,.F.);
#17609=ORIENTED_EDGE('',*,*,#13670,.F.);
#17610=ORIENTED_EDGE('',*,*,#13671,.T.);
#17611=ORIENTED_EDGE('',*,*,#13672,.F.);
#17612=ORIENTED_EDGE('',*,*,#13673,.T.);
#17613=ORIENTED_EDGE('',*,*,#13666,.F.);
#17614=ORIENTED_EDGE('',*,*,#13674,.T.);
#17615=ORIENTED_EDGE('',*,*,#13658,.F.);
#17616=ORIENTED_EDGE('',*,*,#13659,.F.);
#17617=ORIENTED_EDGE('',*,*,#13674,.F.);
#17618=ORIENTED_EDGE('',*,*,#13675,.T.);
#17619=ORIENTED_EDGE('',*,*,#13668,.F.);
#17620=ORIENTED_EDGE('',*,*,#13669,.F.);
#17621=ORIENTED_EDGE('',*,*,#13675,.F.);
#17622=ORIENTED_EDGE('',*,*,#13676,.T.);
#17623=ORIENTED_EDGE('',*,*,#13677,.T.);
#17624=ORIENTED_EDGE('',*,*,#13678,.T.);
#17625=ORIENTED_EDGE('',*,*,#13677,.F.);
#17626=ORIENTED_EDGE('',*,*,#13676,.F.);
#17627=ORIENTED_EDGE('',*,*,#13679,.T.);
#17628=ORIENTED_EDGE('',*,*,#13680,.T.);
#17629=ORIENTED_EDGE('',*,*,#13681,.T.);
#17630=ORIENTED_EDGE('',*,*,#13679,.F.);
#17631=ORIENTED_EDGE('',*,*,#13682,.F.);
#17632=ORIENTED_EDGE('',*,*,#13683,.T.);
#17633=ORIENTED_EDGE('',*,*,#13684,.F.);
#17634=ORIENTED_EDGE('',*,*,#13685,.T.);
#17635=ORIENTED_EDGE('',*,*,#13678,.F.);
#17636=ORIENTED_EDGE('',*,*,#13686,.T.);
#17637=ORIENTED_EDGE('',*,*,#13687,.T.);
#17638=ORIENTED_EDGE('',*,*,#13688,.T.);
#17639=ORIENTED_EDGE('',*,*,#13687,.F.);
#17640=ORIENTED_EDGE('',*,*,#13686,.F.);
#17641=ORIENTED_EDGE('',*,*,#13689,.T.);
#17642=ORIENTED_EDGE('',*,*,#13690,.T.);
#17643=ORIENTED_EDGE('',*,*,#13691,.T.);
#17644=ORIENTED_EDGE('',*,*,#13689,.F.);
#17645=ORIENTED_EDGE('',*,*,#13692,.F.);
#17646=ORIENTED_EDGE('',*,*,#13693,.F.);
#17647=ORIENTED_EDGE('',*,*,#13694,.F.);
#17648=ORIENTED_EDGE('',*,*,#13695,.T.);
#17649=ORIENTED_EDGE('',*,*,#13688,.F.);
#17650=ORIENTED_EDGE('',*,*,#13696,.T.);
#17651=ORIENTED_EDGE('',*,*,#13680,.F.);
#17652=ORIENTED_EDGE('',*,*,#13681,.F.);
#17653=ORIENTED_EDGE('',*,*,#13696,.F.);
#17654=ORIENTED_EDGE('',*,*,#13697,.T.);
#17655=ORIENTED_EDGE('',*,*,#13690,.F.);
#17656=ORIENTED_EDGE('',*,*,#13691,.F.);
#17657=ORIENTED_EDGE('',*,*,#13697,.F.);
#17658=ORIENTED_EDGE('',*,*,#13698,.F.);
#17659=ORIENTED_EDGE('',*,*,#13699,.T.);
#17660=ORIENTED_EDGE('',*,*,#13700,.F.);
#17661=ORIENTED_EDGE('',*,*,#13699,.F.);
#17662=ORIENTED_EDGE('',*,*,#13701,.F.);
#17663=ORIENTED_EDGE('',*,*,#13702,.T.);
#17664=ORIENTED_EDGE('',*,*,#13703,.F.);
#17665=ORIENTED_EDGE('',*,*,#13702,.F.);
#17666=ORIENTED_EDGE('',*,*,#13704,.F.);
#17667=ORIENTED_EDGE('',*,*,#13705,.T.);
#17668=ORIENTED_EDGE('',*,*,#13706,.F.);
#17669=ORIENTED_EDGE('',*,*,#13705,.F.);
#17670=ORIENTED_EDGE('',*,*,#13707,.F.);
#17671=ORIENTED_EDGE('',*,*,#13708,.T.);
#17672=ORIENTED_EDGE('',*,*,#13709,.F.);
#17673=ORIENTED_EDGE('',*,*,#13708,.F.);
#17674=ORIENTED_EDGE('',*,*,#13710,.T.);
#17675=ORIENTED_EDGE('',*,*,#13711,.T.);
#17676=ORIENTED_EDGE('',*,*,#13712,.T.);
#17677=ORIENTED_EDGE('',*,*,#13711,.F.);
#17678=ORIENTED_EDGE('',*,*,#13713,.F.);
#17679=ORIENTED_EDGE('',*,*,#13714,.F.);
#17680=ORIENTED_EDGE('',*,*,#13715,.F.);
#17681=ORIENTED_EDGE('',*,*,#13716,.F.);
#17682=ORIENTED_EDGE('',*,*,#13717,.F.);
#17683=ORIENTED_EDGE('',*,*,#13718,.F.);
#17684=ORIENTED_EDGE('',*,*,#13719,.F.);
#17685=ORIENTED_EDGE('',*,*,#13720,.F.);
#17686=ORIENTED_EDGE('',*,*,#13721,.F.);
#17687=ORIENTED_EDGE('',*,*,#13722,.F.);
#17688=ORIENTED_EDGE('',*,*,#13723,.F.);
#17689=ORIENTED_EDGE('',*,*,#13724,.F.);
#17690=ORIENTED_EDGE('',*,*,#13725,.F.);
#17691=ORIENTED_EDGE('',*,*,#13726,.F.);
#17692=ORIENTED_EDGE('',*,*,#13727,.F.);
#17693=ORIENTED_EDGE('',*,*,#13728,.F.);
#17694=ORIENTED_EDGE('',*,*,#13729,.F.);
#17695=ORIENTED_EDGE('',*,*,#13730,.F.);
#17696=ORIENTED_EDGE('',*,*,#13731,.F.);
#17697=ORIENTED_EDGE('',*,*,#13732,.F.);
#17698=ORIENTED_EDGE('',*,*,#13712,.F.);
#17699=ORIENTED_EDGE('',*,*,#13733,.F.);
#17700=ORIENTED_EDGE('',*,*,#13734,.F.);
#17701=ORIENTED_EDGE('',*,*,#13735,.F.);
#17702=ORIENTED_EDGE('',*,*,#13736,.F.);
#17703=ORIENTED_EDGE('',*,*,#13707,.T.);
#17704=ORIENTED_EDGE('',*,*,#13704,.T.);
#17705=ORIENTED_EDGE('',*,*,#13701,.T.);
#17706=ORIENTED_EDGE('',*,*,#13698,.T.);
#17707=ORIENTED_EDGE('',*,*,#13710,.F.);
#17708=ORIENTED_EDGE('',*,*,#13737,.T.);
#17709=ORIENTED_EDGE('',*,*,#13738,.F.);
#17710=ORIENTED_EDGE('',*,*,#13737,.F.);
#17711=ORIENTED_EDGE('',*,*,#13739,.T.);
#17712=ORIENTED_EDGE('',*,*,#13740,.T.);
#17713=ORIENTED_EDGE('',*,*,#13736,.T.);
#17714=ORIENTED_EDGE('',*,*,#13740,.F.);
#17715=ORIENTED_EDGE('',*,*,#13739,.F.);
#17716=ORIENTED_EDGE('',*,*,#13741,.T.);
#17717=ORIENTED_EDGE('',*,*,#13742,.F.);
#17718=ORIENTED_EDGE('',*,*,#13741,.F.);
#17719=ORIENTED_EDGE('',*,*,#13743,.T.);
#17720=ORIENTED_EDGE('',*,*,#13744,.T.);
#17721=ORIENTED_EDGE('',*,*,#13733,.T.);
#17722=ORIENTED_EDGE('',*,*,#13744,.F.);
#17723=ORIENTED_EDGE('',*,*,#13743,.F.);
#17724=ORIENTED_EDGE('',*,*,#13745,.T.);
#17725=ORIENTED_EDGE('',*,*,#13746,.F.);
#17726=ORIENTED_EDGE('',*,*,#13745,.F.);
#17727=ORIENTED_EDGE('',*,*,#13747,.T.);
#17728=ORIENTED_EDGE('',*,*,#13748,.T.);
#17729=ORIENTED_EDGE('',*,*,#13735,.T.);
#17730=ORIENTED_EDGE('',*,*,#13748,.F.);
#17731=ORIENTED_EDGE('',*,*,#13747,.F.);
#17732=ORIENTED_EDGE('',*,*,#13749,.T.);
#17733=ORIENTED_EDGE('',*,*,#13750,.F.);
#17734=ORIENTED_EDGE('',*,*,#13749,.F.);
#17735=ORIENTED_EDGE('',*,*,#13751,.T.);
#17736=ORIENTED_EDGE('',*,*,#13752,.T.);
#17737=ORIENTED_EDGE('',*,*,#13734,.T.);
#17738=ORIENTED_EDGE('',*,*,#13752,.F.);
#17739=ORIENTED_EDGE('',*,*,#13751,.F.);
#17740=ORIENTED_EDGE('',*,*,#13753,.T.);
#17741=ORIENTED_EDGE('',*,*,#13754,.F.);
#17742=ORIENTED_EDGE('',*,*,#13753,.F.);
#17743=ORIENTED_EDGE('',*,*,#13723,.T.);
#17744=ORIENTED_EDGE('',*,*,#13755,.T.);
#17745=ORIENTED_EDGE('',*,*,#13756,.T.);
#17746=ORIENTED_EDGE('',*,*,#13757,.T.);
#17747=ORIENTED_EDGE('',*,*,#13722,.T.);
#17748=ORIENTED_EDGE('',*,*,#13758,.T.);
#17749=ORIENTED_EDGE('',*,*,#13759,.T.);
#17750=ORIENTED_EDGE('',*,*,#13755,.F.);
#17751=ORIENTED_EDGE('',*,*,#13721,.T.);
#17752=ORIENTED_EDGE('',*,*,#13760,.T.);
#17753=ORIENTED_EDGE('',*,*,#13670,.T.);
#17754=ORIENTED_EDGE('',*,*,#13758,.F.);
#17755=ORIENTED_EDGE('',*,*,#13761,.T.);
#17756=ORIENTED_EDGE('',*,*,#13762,.T.);
#17757=ORIENTED_EDGE('',*,*,#13729,.T.);
#17758=ORIENTED_EDGE('',*,*,#13763,.T.);
#17759=ORIENTED_EDGE('',*,*,#13720,.T.);
#17760=ORIENTED_EDGE('',*,*,#13764,.T.);
#17761=ORIENTED_EDGE('',*,*,#13765,.T.);
#17762=ORIENTED_EDGE('',*,*,#13760,.F.);
#17763=ORIENTED_EDGE('',*,*,#13718,.T.);
#17764=ORIENTED_EDGE('',*,*,#13766,.T.);
#17765=ORIENTED_EDGE('',*,*,#13767,.T.);
#17766=ORIENTED_EDGE('',*,*,#13768,.T.);
#17767=ORIENTED_EDGE('',*,*,#13717,.T.);
#17768=ORIENTED_EDGE('',*,*,#13769,.T.);
#17769=ORIENTED_EDGE('',*,*,#13660,.T.);
#17770=ORIENTED_EDGE('',*,*,#13766,.F.);
#17771=ORIENTED_EDGE('',*,*,#13770,.T.);
#17772=ORIENTED_EDGE('',*,*,#13771,.T.);
#17773=ORIENTED_EDGE('',*,*,#13713,.T.);
#17774=ORIENTED_EDGE('',*,*,#13772,.T.);
#17775=ORIENTED_EDGE('',*,*,#13716,.T.);
#17776=ORIENTED_EDGE('',*,*,#13773,.T.);
#17777=ORIENTED_EDGE('',*,*,#13774,.T.);
#17778=ORIENTED_EDGE('',*,*,#13769,.F.);
#17779=ORIENTED_EDGE('',*,*,#13775,.T.);
#17780=ORIENTED_EDGE('',*,*,#13776,.T.);
#17781=ORIENTED_EDGE('',*,*,#13714,.T.);
#17782=ORIENTED_EDGE('',*,*,#13771,.F.);
#17783=ORIENTED_EDGE('',*,*,#13715,.T.);
#17784=ORIENTED_EDGE('',*,*,#13776,.F.);
#17785=ORIENTED_EDGE('',*,*,#13777,.T.);
#17786=ORIENTED_EDGE('',*,*,#13773,.F.);
#17787=ORIENTED_EDGE('',*,*,#13778,.T.);
#17788=ORIENTED_EDGE('',*,*,#13772,.F.);
#17789=ORIENTED_EDGE('',*,*,#13732,.T.);
#17790=ORIENTED_EDGE('',*,*,#13779,.T.);
#17791=ORIENTED_EDGE('',*,*,#13682,.T.);
#17792=ORIENTED_EDGE('',*,*,#13779,.F.);
#17793=ORIENTED_EDGE('',*,*,#13731,.T.);
#17794=ORIENTED_EDGE('',*,*,#13780,.T.);
#17795=ORIENTED_EDGE('',*,*,#13719,.T.);
#17796=ORIENTED_EDGE('',*,*,#13768,.F.);
#17797=ORIENTED_EDGE('',*,*,#13781,.T.);
#17798=ORIENTED_EDGE('',*,*,#13764,.F.);
#17799=ORIENTED_EDGE('',*,*,#13782,.T.);
#17800=ORIENTED_EDGE('',*,*,#13780,.F.);
#17801=ORIENTED_EDGE('',*,*,#13730,.T.);
#17802=ORIENTED_EDGE('',*,*,#13762,.F.);
#17803=ORIENTED_EDGE('',*,*,#13783,.T.);
#17804=ORIENTED_EDGE('',*,*,#13763,.F.);
#17805=ORIENTED_EDGE('',*,*,#13728,.T.);
#17806=ORIENTED_EDGE('',*,*,#13784,.T.);
#17807=ORIENTED_EDGE('',*,*,#13692,.T.);
#17808=ORIENTED_EDGE('',*,*,#13784,.F.);
#17809=ORIENTED_EDGE('',*,*,#13727,.T.);
#17810=ORIENTED_EDGE('',*,*,#13785,.T.);
#17811=ORIENTED_EDGE('',*,*,#13786,.T.);
#17812=ORIENTED_EDGE('',*,*,#13785,.F.);
#17813=ORIENTED_EDGE('',*,*,#13726,.T.);
#17814=ORIENTED_EDGE('',*,*,#13787,.T.);
#17815=ORIENTED_EDGE('',*,*,#13724,.T.);
#17816=ORIENTED_EDGE('',*,*,#13757,.F.);
#17817=ORIENTED_EDGE('',*,*,#13788,.T.);
#17818=ORIENTED_EDGE('',*,*,#13789,.T.);
#17819=ORIENTED_EDGE('',*,*,#13725,.T.);
#17820=ORIENTED_EDGE('',*,*,#13789,.F.);
#17821=ORIENTED_EDGE('',*,*,#13790,.T.);
#17822=ORIENTED_EDGE('',*,*,#13787,.F.);
#17823=ORIENTED_EDGE('',*,*,#13759,.F.);
#17824=ORIENTED_EDGE('',*,*,#13673,.F.);
#17825=ORIENTED_EDGE('',*,*,#13791,.F.);
#17826=ORIENTED_EDGE('',*,*,#13792,.T.);
#17827=ORIENTED_EDGE('',*,*,#13765,.F.);
#17828=ORIENTED_EDGE('',*,*,#13793,.F.);
#17829=ORIENTED_EDGE('',*,*,#13794,.F.);
#17830=ORIENTED_EDGE('',*,*,#13671,.F.);
#17831=ORIENTED_EDGE('',*,*,#13781,.F.);
#17832=ORIENTED_EDGE('',*,*,#13795,.F.);
#17833=ORIENTED_EDGE('',*,*,#13796,.F.);
#17834=ORIENTED_EDGE('',*,*,#13793,.T.);
#17835=ORIENTED_EDGE('',*,*,#13767,.F.);
#17836=ORIENTED_EDGE('',*,*,#13663,.F.);
#17837=ORIENTED_EDGE('',*,*,#13797,.F.);
#17838=ORIENTED_EDGE('',*,*,#13795,.T.);
#17839=ORIENTED_EDGE('',*,*,#13774,.F.);
#17840=ORIENTED_EDGE('',*,*,#13798,.T.);
#17841=ORIENTED_EDGE('',*,*,#13799,.F.);
#17842=ORIENTED_EDGE('',*,*,#13661,.T.);
#17843=ORIENTED_EDGE('',*,*,#13777,.F.);
#17844=ORIENTED_EDGE('',*,*,#13800,.F.);
#17845=ORIENTED_EDGE('',*,*,#13801,.F.);
#17846=ORIENTED_EDGE('',*,*,#13798,.F.);
#17847=ORIENTED_EDGE('',*,*,#13775,.F.);
#17848=ORIENTED_EDGE('',*,*,#13802,.F.);
#17849=ORIENTED_EDGE('',*,*,#13803,.F.);
#17850=ORIENTED_EDGE('',*,*,#13800,.T.);
#17851=ORIENTED_EDGE('',*,*,#13770,.F.);
#17852=ORIENTED_EDGE('',*,*,#13804,.F.);
#17853=ORIENTED_EDGE('',*,*,#13805,.F.);
#17854=ORIENTED_EDGE('',*,*,#13802,.T.);
#17855=ORIENTED_EDGE('',*,*,#13790,.F.);
#17856=ORIENTED_EDGE('',*,*,#13806,.F.);
#17857=ORIENTED_EDGE('',*,*,#13807,.F.);
#17858=ORIENTED_EDGE('',*,*,#13808,.F.);
#17859=ORIENTED_EDGE('',*,*,#13756,.F.);
#17860=ORIENTED_EDGE('',*,*,#13792,.F.);
#17861=ORIENTED_EDGE('',*,*,#13809,.F.);
#17862=ORIENTED_EDGE('',*,*,#13810,.T.);
#17863=ORIENTED_EDGE('',*,*,#13788,.F.);
#17864=ORIENTED_EDGE('',*,*,#13810,.F.);
#17865=ORIENTED_EDGE('',*,*,#13811,.F.);
#17866=ORIENTED_EDGE('',*,*,#13806,.T.);
#17867=ORIENTED_EDGE('',*,*,#13778,.F.);
#17868=ORIENTED_EDGE('',*,*,#13685,.F.);
#17869=ORIENTED_EDGE('',*,*,#13812,.F.);
#17870=ORIENTED_EDGE('',*,*,#13804,.T.);
#17871=ORIENTED_EDGE('',*,*,#13786,.F.);
#17872=ORIENTED_EDGE('',*,*,#13808,.T.);
#17873=ORIENTED_EDGE('',*,*,#13813,.F.);
#17874=ORIENTED_EDGE('',*,*,#13693,.T.);
#17875=ORIENTED_EDGE('',*,*,#13801,.T.);
#17876=ORIENTED_EDGE('',*,*,#13803,.T.);
#17877=ORIENTED_EDGE('',*,*,#13805,.T.);
#17878=ORIENTED_EDGE('',*,*,#13812,.T.);
#17879=ORIENTED_EDGE('',*,*,#13684,.T.);
#17880=ORIENTED_EDGE('',*,*,#13814,.T.);
#17881=ORIENTED_EDGE('',*,*,#13815,.T.);
#17882=ORIENTED_EDGE('',*,*,#13816,.T.);
#17883=ORIENTED_EDGE('',*,*,#13694,.T.);
#17884=ORIENTED_EDGE('',*,*,#13813,.T.);
#17885=ORIENTED_EDGE('',*,*,#13807,.T.);
#17886=ORIENTED_EDGE('',*,*,#13811,.T.);
#17887=ORIENTED_EDGE('',*,*,#13809,.T.);
#17888=ORIENTED_EDGE('',*,*,#13791,.T.);
#17889=ORIENTED_EDGE('',*,*,#13672,.T.);
#17890=ORIENTED_EDGE('',*,*,#13794,.T.);
#17891=ORIENTED_EDGE('',*,*,#13796,.T.);
#17892=ORIENTED_EDGE('',*,*,#13797,.T.);
#17893=ORIENTED_EDGE('',*,*,#13662,.T.);
#17894=ORIENTED_EDGE('',*,*,#13799,.T.);
#17895=ORIENTED_EDGE('',*,*,#13750,.T.);
#17896=ORIENTED_EDGE('',*,*,#13746,.T.);
#17897=ORIENTED_EDGE('',*,*,#13742,.T.);
#17898=ORIENTED_EDGE('',*,*,#13738,.T.);
#17899=ORIENTED_EDGE('',*,*,#13754,.T.);
#17900=ORIENTED_EDGE('',*,*,#13709,.T.);
#17901=ORIENTED_EDGE('',*,*,#13706,.T.);
#17902=ORIENTED_EDGE('',*,*,#13703,.T.);
#17903=ORIENTED_EDGE('',*,*,#13700,.T.);
#17904=ORIENTED_EDGE('',*,*,#13761,.F.);
#17905=ORIENTED_EDGE('',*,*,#13817,.F.);
#17906=ORIENTED_EDGE('',*,*,#13815,.F.);
#17907=ORIENTED_EDGE('',*,*,#13818,.T.);
#17908=ORIENTED_EDGE('',*,*,#13782,.F.);
#17909=ORIENTED_EDGE('',*,*,#13818,.F.);
#17910=ORIENTED_EDGE('',*,*,#13814,.F.);
#17911=ORIENTED_EDGE('',*,*,#13683,.F.);
#17912=ORIENTED_EDGE('',*,*,#13783,.F.);
#17913=ORIENTED_EDGE('',*,*,#13695,.F.);
#17914=ORIENTED_EDGE('',*,*,#13816,.F.);
#17915=ORIENTED_EDGE('',*,*,#13817,.T.);
#25450=CONICAL_SURFACE('',#27100,1.9525,0.785398163397448);
#25451=CONICAL_SURFACE('',#27107,1.9525,0.785398163397448);
#25452=CONICAL_SURFACE('',#27114,1.80249999999999,1.02974425867665);
#25453=CONICAL_SURFACE('',#27115,1.80249999999999,1.02974425867665);
#25454=CONICAL_SURFACE('',#27116,1.9525,0.785398163397448);
#25455=CONICAL_SURFACE('',#27123,1.9525,0.785398163397448);
#25456=CONICAL_SURFACE('',#27130,0.901249999999996,1.02974425867665);
#25457=CONICAL_SURFACE('',#27131,0.901249999999996,1.02974425867665);
#25458=CONICAL_SURFACE('',#27144,1.9525,0.785398163397445);
#25459=CONICAL_SURFACE('',#27154,1.9525,0.785398163397444);
#25460=CONICAL_SURFACE('',#27158,1.9525,0.785398163397444);
#25461=CONICAL_SURFACE('',#27162,1.9525,0.785398163397445);
#25462=CONICAL_SURFACE('',#27166,6.563,0.785398163397448);
#25550=ADVANCED_FACE('',(#2357),#25450,.F.);
#25551=ADVANCED_FACE('',(#2358),#2142,.F.);
#25552=ADVANCED_FACE('',(#2359,#961),#1123,.T.);
#25553=ADVANCED_FACE('',(#2360),#25451,.F.);
#25554=ADVANCED_FACE('',(#2361),#2143,.F.);
#25555=ADVANCED_FACE('',(#2362,#962),#1124,.T.);
#25556=ADVANCED_FACE('',(#2363),#25452,.F.);
#25557=ADVANCED_FACE('',(#2364),#25453,.F.);
#25558=ADVANCED_FACE('',(#2365),#25454,.F.);
#25559=ADVANCED_FACE('',(#2366),#2144,.F.);
#25560=ADVANCED_FACE('',(#2367,#963),#1125,.T.);
#25561=ADVANCED_FACE('',(#2368),#25455,.F.);
#25562=ADVANCED_FACE('',(#2369),#2145,.F.);
#25563=ADVANCED_FACE('',(#2370,#964),#1126,.T.);
#25564=ADVANCED_FACE('',(#2371),#25456,.F.);
#25565=ADVANCED_FACE('',(#2372),#25457,.F.);
#25566=ADVANCED_FACE('',(#2373),#2146,.F.);
#25567=ADVANCED_FACE('',(#2374),#2147,.F.);
#25568=ADVANCED_FACE('',(#2375),#2148,.F.);
#25569=ADVANCED_FACE('',(#2376),#2149,.F.);
#25570=ADVANCED_FACE('',(#2377),#25458,.F.);
#25571=ADVANCED_FACE('',(#2378,#965,#966,#967,#968,#969,#970,#971,#972,
#973),#1127,.T.);
#25572=ADVANCED_FACE('',(#2379),#2150,.F.);
#25573=ADVANCED_FACE('',(#2380),#25459,.F.);
#25574=ADVANCED_FACE('',(#2381),#2151,.F.);
#25575=ADVANCED_FACE('',(#2382),#25460,.F.);
#25576=ADVANCED_FACE('',(#2383),#2152,.F.);
#25577=ADVANCED_FACE('',(#2384),#25461,.F.);
#25578=ADVANCED_FACE('',(#2385),#2153,.F.);
#25579=ADVANCED_FACE('',(#2386),#25462,.F.);
#25580=ADVANCED_FACE('',(#2387),#2154,.F.);
#25581=ADVANCED_FACE('',(#2388),#1128,.T.);
#25582=ADVANCED_FACE('',(#2389),#1129,.T.);
#25583=ADVANCED_FACE('',(#2390),#1130,.T.);
#25584=ADVANCED_FACE('',(#2391),#1131,.T.);
#25585=ADVANCED_FACE('',(#2392),#1132,.T.);
#25586=ADVANCED_FACE('',(#2393),#1133,.T.);
#25587=ADVANCED_FACE('',(#2394),#1134,.T.);
#25588=ADVANCED_FACE('',(#2395),#1135,.T.);
#25589=ADVANCED_FACE('',(#2396),#1136,.T.);
#25590=ADVANCED_FACE('',(#2397),#1137,.T.);
#25591=ADVANCED_FACE('',(#2398),#1138,.T.);
#25592=ADVANCED_FACE('',(#2399),#1139,.T.);
#25593=ADVANCED_FACE('',(#2400),#1140,.T.);
#25594=ADVANCED_FACE('',(#2401),#1141,.T.);
#25595=ADVANCED_FACE('',(#2402),#1142,.T.);
#25596=ADVANCED_FACE('',(#2403),#1143,.T.);
#25597=ADVANCED_FACE('',(#2404),#1144,.T.);
#25598=ADVANCED_FACE('',(#2405),#1145,.T.);
#25599=ADVANCED_FACE('',(#2406),#1146,.T.);
#25600=ADVANCED_FACE('',(#2407),#1147,.T.);
#25601=ADVANCED_FACE('',(#2408),#1148,.T.);
#25602=ADVANCED_FACE('',(#2409),#1149,.F.);
#25603=ADVANCED_FACE('',(#2410),#1150,.F.);
#25604=ADVANCED_FACE('',(#2411),#1151,.F.);
#25605=ADVANCED_FACE('',(#2412),#1152,.T.);
#25606=ADVANCED_FACE('',(#2413),#1153,.F.);
#25607=ADVANCED_FACE('',(#2414),#1154,.F.);
#25608=ADVANCED_FACE('',(#2415),#1155,.F.);
#25609=ADVANCED_FACE('',(#2416),#1156,.F.);
#25610=ADVANCED_FACE('',(#2417),#1157,.F.);
#25611=ADVANCED_FACE('',(#2418),#1158,.F.);
#25612=ADVANCED_FACE('',(#2419),#1159,.T.);
#25613=ADVANCED_FACE('',(#2420),#1160,.T.);
#25614=ADVANCED_FACE('',(#2421,#974,#975,#976,#977,#978,#979,#980,#981,
#982),#1161,.F.);
#25615=ADVANCED_FACE('',(#2422),#1162,.F.);
#25616=ADVANCED_FACE('',(#2423),#1163,.F.);
#25617=ADVANCED_FACE('',(#2424),#1164,.F.);
#26929=CLOSED_SHELL('',(#25550,#25551,#25552,#25553,#25554,#25555,#25556,
#25557,#25558,#25559,#25560,#25561,#25562,#25563,#25564,#25565,#25566,#25567,
#25568,#25569,#25570,#25571,#25572,#25573,#25574,#25575,#25576,#25577,#25578,
#25579,#25580,#25581,#25582,#25583,#25584,#25585,#25586,#25587,#25588,#25589,
#25590,#25591,#25592,#25593,#25594,#25595,#25596,#25597,#25598,#25599,#25600,
#25601,#25602,#25603,#25604,#25605,#25606,#25607,#25608,#25609,#25610,#25611,
#25612,#25613,#25614,#25615,#25616,#25617));
#27099=AXIS2_PLACEMENT_3D('',#36081,#29257,#29258);
#27100=AXIS2_PLACEMENT_3D('',#36082,#29259,#29260);
#27101=AXIS2_PLACEMENT_3D('',#36084,#29261,#29262);
#27102=AXIS2_PLACEMENT_3D('',#36087,#29264,#29265);
#27103=AXIS2_PLACEMENT_3D('',#36088,#29266,#29267);
#27104=AXIS2_PLACEMENT_3D('',#36092,#29269,#29270);
#27105=AXIS2_PLACEMENT_3D('',#36093,#29271,#29272);
#27106=AXIS2_PLACEMENT_3D('',#36094,#29273,#29274);
#27107=AXIS2_PLACEMENT_3D('',#36103,#29279,#29280);
#27108=AXIS2_PLACEMENT_3D('',#36105,#29281,#29282);
#27109=AXIS2_PLACEMENT_3D('',#36108,#29284,#29285);
#27110=AXIS2_PLACEMENT_3D('',#36109,#29286,#29287);
#27111=AXIS2_PLACEMENT_3D('',#36113,#29289,#29290);
#27112=AXIS2_PLACEMENT_3D('',#36114,#29291,#29292);
#27113=AXIS2_PLACEMENT_3D('',#36115,#29293,#29294);
#27114=AXIS2_PLACEMENT_3D('',#36124,#29299,#29300);
#27115=AXIS2_PLACEMENT_3D('',#36127,#29302,#29303);
#27116=AXIS2_PLACEMENT_3D('',#36130,#29305,#29306);
#27117=AXIS2_PLACEMENT_3D('',#36132,#29307,#29308);
#27118=AXIS2_PLACEMENT_3D('',#36135,#29310,#29311);
#27119=AXIS2_PLACEMENT_3D('',#36136,#29312,#29313);
#27120=AXIS2_PLACEMENT_3D('',#36140,#29315,#29316);
#27121=AXIS2_PLACEMENT_3D('',#36141,#29317,#29318);
#27122=AXIS2_PLACEMENT_3D('',#36142,#29319,#29320);
#27123=AXIS2_PLACEMENT_3D('',#36151,#29325,#29326);
#27124=AXIS2_PLACEMENT_3D('',#36153,#29327,#29328);
#27125=AXIS2_PLACEMENT_3D('',#36156,#29330,#29331);
#27126=AXIS2_PLACEMENT_3D('',#36157,#29332,#29333);
#27127=AXIS2_PLACEMENT_3D('',#36161,#29335,#29336);
#27128=AXIS2_PLACEMENT_3D('',#36162,#29337,#29338);
#27129=AXIS2_PLACEMENT_3D('',#36163,#29339,#29340);
#27130=AXIS2_PLACEMENT_3D('',#36172,#29345,#29346);
#27131=AXIS2_PLACEMENT_3D('',#36175,#29348,#29349);
#27132=AXIS2_PLACEMENT_3D('',#36178,#29351,#29352);
#27133=AXIS2_PLACEMENT_3D('',#36180,#29353,#29354);
#27134=AXIS2_PLACEMENT_3D('',#36183,#29356,#29357);
#27135=AXIS2_PLACEMENT_3D('',#36184,#29358,#29359);
#27136=AXIS2_PLACEMENT_3D('',#36186,#29360,#29361);
#27137=AXIS2_PLACEMENT_3D('',#36189,#29363,#29364);
#27138=AXIS2_PLACEMENT_3D('',#36190,#29365,#29366);
#27139=AXIS2_PLACEMENT_3D('',#36192,#29367,#29368);
#27140=AXIS2_PLACEMENT_3D('',#36195,#29370,#29371);
#27141=AXIS2_PLACEMENT_3D('',#36196,#29372,#29373);
#27142=AXIS2_PLACEMENT_3D('',#36198,#29374,#29375);
#27143=AXIS2_PLACEMENT_3D('',#36201,#29377,#29378);
#27144=AXIS2_PLACEMENT_3D('',#36202,#29379,#29380);
#27145=AXIS2_PLACEMENT_3D('',#36204,#29381,#29382);
#27146=AXIS2_PLACEMENT_3D('',#36207,#29384,#29385);
#27147=AXIS2_PLACEMENT_3D('',#36208,#29386,#29387);
#27148=AXIS2_PLACEMENT_3D('',#36250,#29408,#29409);
#27149=AXIS2_PLACEMENT_3D('',#36252,#29410,#29411);
#27150=AXIS2_PLACEMENT_3D('',#36254,#29412,#29413);
#27151=AXIS2_PLACEMENT_3D('',#36256,#29414,#29415);
#27152=AXIS2_PLACEMENT_3D('',#36257,#29416,#29417);
#27153=AXIS2_PLACEMENT_3D('',#36260,#29419,#29420);
#27154=AXIS2_PLACEMENT_3D('',#36261,#29421,#29422);
#27155=AXIS2_PLACEMENT_3D('',#36263,#29423,#29424);
#27156=AXIS2_PLACEMENT_3D('',#36265,#29426,#29427);
#27157=AXIS2_PLACEMENT_3D('',#36268,#29429,#29430);
#27158=AXIS2_PLACEMENT_3D('',#36269,#29431,#29432);
#27159=AXIS2_PLACEMENT_3D('',#36271,#29433,#29434);
#27160=AXIS2_PLACEMENT_3D('',#36273,#29436,#29437);
#27161=AXIS2_PLACEMENT_3D('',#36276,#29439,#29440);
#27162=AXIS2_PLACEMENT_3D('',#36277,#29441,#29442);
#27163=AXIS2_PLACEMENT_3D('',#36279,#29443,#29444);
#27164=AXIS2_PLACEMENT_3D('',#36281,#29446,#29447);
#27165=AXIS2_PLACEMENT_3D('',#36284,#29449,#29450);
#27166=AXIS2_PLACEMENT_3D('',#36285,#29451,#29452);
#27167=AXIS2_PLACEMENT_3D('',#36287,#29453,#29454);
#27168=AXIS2_PLACEMENT_3D('',#36289,#29456,#29457);
#27169=AXIS2_PLACEMENT_3D('',#36292,#29459,#29460);
#27170=AXIS2_PLACEMENT_3D('',#36293,#29461,#29462);
#27171=AXIS2_PLACEMENT_3D('',#36299,#29466,#29467);
#27172=AXIS2_PLACEMENT_3D('',#36302,#29470,#29471);
#27173=AXIS2_PLACEMENT_3D('',#36304,#29473,#29474);
#27174=AXIS2_PLACEMENT_3D('',#36310,#29478,#29479);
#27175=AXIS2_PLACEMENT_3D('',#36314,#29482,#29483);
#27176=AXIS2_PLACEMENT_3D('',#36319,#29487,#29488);
#27177=AXIS2_PLACEMENT_3D('',#36321,#29490,#29491);
#27178=AXIS2_PLACEMENT_3D('',#36327,#29495,#29496);
#27179=AXIS2_PLACEMENT_3D('',#36331,#29499,#29500);
#27180=AXIS2_PLACEMENT_3D('',#36335,#29503,#29504);
#27181=AXIS2_PLACEMENT_3D('',#36337,#29506,#29507);
#27182=AXIS2_PLACEMENT_3D('',#36340,#29510,#29511);
#27183=AXIS2_PLACEMENT_3D('',#36342,#29513,#29514);
#27184=AXIS2_PLACEMENT_3D('',#36344,#29516,#29517);
#27185=AXIS2_PLACEMENT_3D('',#36346,#29519,#29520);
#27186=AXIS2_PLACEMENT_3D('',#36349,#29523,#29524);
#27187=AXIS2_PLACEMENT_3D('',#36351,#29526,#29527);
#27188=AXIS2_PLACEMENT_3D('',#36355,#29530,#29531);
#27189=AXIS2_PLACEMENT_3D('',#36359,#29534,#29535);
#27190=AXIS2_PLACEMENT_3D('',#36361,#29537,#29538);
#27191=AXIS2_PLACEMENT_3D('',#36365,#29541,#29542);
#27192=AXIS2_PLACEMENT_3D('',#36369,#29545,#29546);
#27193=AXIS2_PLACEMENT_3D('',#36373,#29549,#29550);
#27194=AXIS2_PLACEMENT_3D('',#36375,#29552,#29553);
#27195=AXIS2_PLACEMENT_3D('',#36379,#29556,#29557);
#27196=AXIS2_PLACEMENT_3D('',#36383,#29560,#29561);
#27197=AXIS2_PLACEMENT_3D('',#36387,#29564,#29565);
#27198=AXIS2_PLACEMENT_3D('',#36391,#29568,#29569);
#27199=AXIS2_PLACEMENT_3D('',#36397,#29573,#29574);
#27200=AXIS2_PLACEMENT_3D('',#36401,#29577,#29578);
#27201=AXIS2_PLACEMENT_3D('',#36403,#29580,#29581);
#27202=AXIS2_PLACEMENT_3D('',#36405,#29583,#29584);
#27203=AXIS2_PLACEMENT_3D('',#36407,#29586,#29587);
#27204=AXIS2_PLACEMENT_3D('',#36413,#29591,#29592);
#27205=AXIS2_PLACEMENT_3D('',#36416,#29595,#29596);
#27206=AXIS2_PLACEMENT_3D('',#36417,#29597,#29598);
#29257=DIRECTION('axis',(0.,0.,1.));
#29258=DIRECTION('refdir',(1.,0.,0.));
#29259=DIRECTION('center_axis',(-1.,0.,0.));
#29260=DIRECTION('ref_axis',(0.,0.,-1.));
#29261=DIRECTION('center_axis',(1.,0.,0.));
#29262=DIRECTION('ref_axis',(0.,0.,-1.));
#29263=DIRECTION('',(-0.707106781186548,8.65956056235493E-17,0.707106781186547));
#29264=DIRECTION('center_axis',(-1.,0.,0.));
#29265=DIRECTION('ref_axis',(0.,0.,-1.));
#29266=DIRECTION('center_axis',(1.,0.,0.));
#29267=DIRECTION('ref_axis',(0.,0.,-1.));
#29268=DIRECTION('',(1.,0.,0.));
#29269=DIRECTION('center_axis',(1.,0.,0.));
#29270=DIRECTION('ref_axis',(0.,0.,-1.));
#29271=DIRECTION('center_axis',(1.,0.,0.));
#29272=DIRECTION('ref_axis',(0.,0.,-1.));
#29273=DIRECTION('center_axis',(-1.,0.,0.));
#29274=DIRECTION('ref_axis',(0.,0.,1.));
#29275=DIRECTION('',(0.,0.,1.));
#29276=DIRECTION('',(0.,1.,0.));
#29277=DIRECTION('',(0.,0.,-1.));
#29278=DIRECTION('',(0.,1.,0.));
#29279=DIRECTION('center_axis',(-1.,0.,0.));
#29280=DIRECTION('ref_axis',(0.,0.,-1.));
#29281=DIRECTION('center_axis',(1.,0.,0.));
#29282=DIRECTION('ref_axis',(0.,0.,-1.));
#29283=DIRECTION('',(-0.707106781186548,8.65956056235493E-17,0.707106781186547));
#29284=DIRECTION('center_axis',(-1.,0.,0.));
#29285=DIRECTION('ref_axis',(0.,0.,-1.));
#29286=DIRECTION('center_axis',(1.,0.,0.));
#29287=DIRECTION('ref_axis',(0.,0.,-1.));
#29288=DIRECTION('',(1.,0.,0.));
#29289=DIRECTION('center_axis',(1.,0.,0.));
#29290=DIRECTION('ref_axis',(0.,0.,-1.));
#29291=DIRECTION('center_axis',(1.,0.,0.));
#29292=DIRECTION('ref_axis',(0.,0.,-1.));
#29293=DIRECTION('center_axis',(-1.,0.,0.));
#29294=DIRECTION('ref_axis',(0.,0.,1.));
#29295=DIRECTION('',(0.,0.,1.));
#29296=DIRECTION('',(0.,-1.,0.));
#29297=DIRECTION('',(0.,0.,-1.));
#29298=DIRECTION('',(0.,1.,0.));
#29299=DIRECTION('center_axis',(-1.,0.,0.));
#29300=DIRECTION('ref_axis',(0.,1.,0.));
#29301=DIRECTION('',(-0.515038074910058,-0.85716730070211,1.04972719113862E-16));
#29302=DIRECTION('center_axis',(-1.,0.,0.));
#29303=DIRECTION('ref_axis',(0.,1.,0.));
#29304=DIRECTION('',(-0.515038074910058,-0.85716730070211,1.04972719113862E-16));
#29305=DIRECTION('center_axis',(1.,0.,0.));
#29306=DIRECTION('ref_axis',(0.,0.,-1.));
#29307=DIRECTION('center_axis',(-1.,0.,0.));
#29308=DIRECTION('ref_axis',(0.,0.,-1.));
#29309=DIRECTION('',(0.707106781186548,-8.65956056235493E-17,0.707106781186547));
#29310=DIRECTION('center_axis',(1.,0.,0.));
#29311=DIRECTION('ref_axis',(0.,0.,-1.));
#29312=DIRECTION('center_axis',(-1.,0.,0.));
#29313=DIRECTION('ref_axis',(0.,0.,-1.));
#29314=DIRECTION('',(-1.,0.,0.));
#29315=DIRECTION('center_axis',(-1.,0.,0.));
#29316=DIRECTION('ref_axis',(0.,0.,-1.));
#29317=DIRECTION('center_axis',(-1.,0.,0.));
#29318=DIRECTION('ref_axis',(0.,0.,-1.));
#29319=DIRECTION('center_axis',(1.,0.,0.));
#29320=DIRECTION('ref_axis',(0.,0.,-1.));
#29321=DIRECTION('',(0.,0.,-1.));
#29322=DIRECTION('',(0.,-1.,0.));
#29323=DIRECTION('',(0.,0.,1.));
#29324=DIRECTION('',(0.,1.,0.));
#29325=DIRECTION('center_axis',(1.,0.,0.));
#29326=DIRECTION('ref_axis',(0.,0.,-1.));
#29327=DIRECTION('center_axis',(-1.,0.,0.));
#29328=DIRECTION('ref_axis',(0.,0.,-1.));
#29329=DIRECTION('',(0.707106781186548,-8.65956056235493E-17,0.707106781186547));
#29330=DIRECTION('center_axis',(1.,0.,0.));
#29331=DIRECTION('ref_axis',(0.,0.,-1.));
#29332=DIRECTION('center_axis',(-1.,0.,0.));
#29333=DIRECTION('ref_axis',(0.,0.,-1.));
#29334=DIRECTION('',(-1.,0.,0.));
#29335=DIRECTION('center_axis',(-1.,0.,0.));
#29336=DIRECTION('ref_axis',(0.,0.,-1.));
#29337=DIRECTION('center_axis',(-1.,0.,0.));
#29338=DIRECTION('ref_axis',(0.,0.,-1.));
#29339=DIRECTION('center_axis',(1.,0.,0.));
#29340=DIRECTION('ref_axis',(0.,0.,-1.));
#29341=DIRECTION('',(0.,0.,-1.));
#29342=DIRECTION('',(0.,1.,0.));
#29343=DIRECTION('',(0.,0.,1.));
#29344=DIRECTION('',(0.,1.,0.));
#29345=DIRECTION('center_axis',(1.,0.,0.));
#29346=DIRECTION('ref_axis',(0.,1.,0.));
#29347=DIRECTION('',(0.515038074910058,-0.85716730070211,-1.04972719113862E-16));
#29348=DIRECTION('center_axis',(1.,0.,0.));
#29349=DIRECTION('ref_axis',(0.,1.,0.));
#29350=DIRECTION('',(0.515038074910058,-0.85716730070211,-1.04972719113862E-16));
#29351=DIRECTION('center_axis',(0.,-1.,0.));
#29352=DIRECTION('ref_axis',(1.,0.,0.));
#29353=DIRECTION('center_axis',(0.,-1.,0.));
#29354=DIRECTION('ref_axis',(1.,0.,0.));
#29355=DIRECTION('',(0.,-1.,0.));
#29356=DIRECTION('center_axis',(0.,1.,0.));
#29357=DIRECTION('ref_axis',(1.,0.,0.));
#29358=DIRECTION('center_axis',(0.,-1.,0.));
#29359=DIRECTION('ref_axis',(1.,0.,0.));
#29360=DIRECTION('center_axis',(0.,-1.,0.));
#29361=DIRECTION('ref_axis',(1.,0.,0.));
#29362=DIRECTION('',(0.,-1.,0.));
#29363=DIRECTION('center_axis',(0.,1.,0.));
#29364=DIRECTION('ref_axis',(1.,0.,0.));
#29365=DIRECTION('center_axis',(0.,-1.,0.));
#29366=DIRECTION('ref_axis',(1.,0.,0.));
#29367=DIRECTION('center_axis',(0.,-1.,0.));
#29368=DIRECTION('ref_axis',(1.,0.,0.));
#29369=DIRECTION('',(0.,-1.,0.));
#29370=DIRECTION('center_axis',(0.,1.,0.));
#29371=DIRECTION('ref_axis',(1.,0.,0.));
#29372=DIRECTION('center_axis',(0.,-1.,0.));
#29373=DIRECTION('ref_axis',(1.,0.,0.));
#29374=DIRECTION('center_axis',(0.,-1.,0.));
#29375=DIRECTION('ref_axis',(1.,0.,0.));
#29376=DIRECTION('',(0.,-1.,0.));
#29377=DIRECTION('center_axis',(0.,1.,0.));
#29378=DIRECTION('ref_axis',(1.,0.,0.));
#29379=DIRECTION('center_axis',(0.,1.,0.));
#29380=DIRECTION('ref_axis',(1.,0.,0.));
#29381=DIRECTION('center_axis',(0.,-1.,0.));
#29382=DIRECTION('ref_axis',(1.,0.,0.));
#29383=DIRECTION('',(-0.707106781186545,0.70710678118655,8.6595605623549E-17));
#29384=DIRECTION('center_axis',(0.,1.,0.));
#29385=DIRECTION('ref_axis',(1.,0.,0.));
#29386=DIRECTION('center_axis',(0.,1.,0.));
#29387=DIRECTION('ref_axis',(0.,0.,1.));
#29388=DIRECTION('',(0.541178323236022,0.,-0.840907856105203));
#29389=DIRECTION('',(1.,0.,0.));
#29390=DIRECTION('',(0.541178323236022,0.,0.840907856105203));
#29391=DIRECTION('',(1.,0.,0.));
#29392=DIRECTION('',(0.,0.,-1.));
#29393=DIRECTION('',(-1.,0.,0.));
#29394=DIRECTION('',(0.,0.,-1.));
#29395=DIRECTION('',(1.,0.,0.));
#29396=DIRECTION('',(0.,0.,-1.));
#29397=DIRECTION('',(-1.,0.,0.));
#29398=DIRECTION('',(-0.541178323236022,0.,0.840907856105203));
#29399=DIRECTION('',(-1.,0.,0.));
#29400=DIRECTION('',(-0.541178323236022,0.,-0.840907856105203));
#29401=DIRECTION('',(-1.,0.,0.));
#29402=DIRECTION('',(0.,0.,1.));
#29403=DIRECTION('',(1.,0.,0.));
#29404=DIRECTION('',(0.,0.,1.));
#29405=DIRECTION('',(-1.,0.,0.));
#29406=DIRECTION('',(0.,0.,1.));
#29407=DIRECTION('',(1.,0.,0.));
#29408=DIRECTION('center_axis',(0.,1.,0.));
#29409=DIRECTION('ref_axis',(1.,0.,0.));
#29410=DIRECTION('center_axis',(0.,1.,0.));
#29411=DIRECTION('ref_axis',(1.,0.,0.));
#29412=DIRECTION('center_axis',(0.,1.,0.));
#29413=DIRECTION('ref_axis',(1.,0.,0.));
#29414=DIRECTION('center_axis',(0.,1.,0.));
#29415=DIRECTION('ref_axis',(1.,0.,0.));
#29416=DIRECTION('center_axis',(0.,-1.,0.));
#29417=DIRECTION('ref_axis',(1.,0.,0.));
#29418=DIRECTION('',(0.,-1.,0.));
#29419=DIRECTION('center_axis',(0.,1.,0.));
#29420=DIRECTION('ref_axis',(1.,0.,0.));
#29421=DIRECTION('center_axis',(0.,1.,0.));
#29422=DIRECTION('ref_axis',(1.,0.,0.));
#29423=DIRECTION('center_axis',(0.,-1.,0.));
#29424=DIRECTION('ref_axis',(1.,0.,0.));
#29425=DIRECTION('',(-0.707106781186545,0.707106781186551,8.65956056235489E-17));
#29426=DIRECTION('center_axis',(0.,-1.,0.));
#29427=DIRECTION('ref_axis',(1.,0.,0.));
#29428=DIRECTION('',(0.,-1.,0.));
#29429=DIRECTION('center_axis',(0.,1.,0.));
#29430=DIRECTION('ref_axis',(1.,0.,0.));
#29431=DIRECTION('center_axis',(0.,1.,0.));
#29432=DIRECTION('ref_axis',(1.,0.,0.));
#29433=DIRECTION('center_axis',(0.,-1.,0.));
#29434=DIRECTION('ref_axis',(1.,0.,0.));
#29435=DIRECTION('',(-0.707106781186545,0.707106781186551,8.65956056235489E-17));
#29436=DIRECTION('center_axis',(0.,-1.,0.));
#29437=DIRECTION('ref_axis',(1.,0.,0.));
#29438=DIRECTION('',(0.,-1.,0.));
#29439=DIRECTION('center_axis',(0.,1.,0.));
#29440=DIRECTION('ref_axis',(1.,0.,0.));
#29441=DIRECTION('center_axis',(0.,1.,0.));
#29442=DIRECTION('ref_axis',(1.,0.,0.));
#29443=DIRECTION('center_axis',(0.,-1.,0.));
#29444=DIRECTION('ref_axis',(1.,0.,0.));
#29445=DIRECTION('',(-0.707106781186545,0.70710678118655,8.6595605623549E-17));
#29446=DIRECTION('center_axis',(0.,-1.,0.));
#29447=DIRECTION('ref_axis',(1.,0.,0.));
#29448=DIRECTION('',(0.,-1.,0.));
#29449=DIRECTION('center_axis',(0.,1.,0.));
#29450=DIRECTION('ref_axis',(1.,0.,0.));
#29451=DIRECTION('center_axis',(0.,1.,0.));
#29452=DIRECTION('ref_axis',(1.,0.,0.));
#29453=DIRECTION('center_axis',(0.,-1.,0.));
#29454=DIRECTION('ref_axis',(1.,0.,0.));
#29455=DIRECTION('',(-0.707106781186547,0.707106781186548,8.65956056235493E-17));
#29456=DIRECTION('center_axis',(0.,-1.,0.));
#29457=DIRECTION('ref_axis',(1.,0.,0.));
#29458=DIRECTION('',(0.,-1.,0.));
#29459=DIRECTION('center_axis',(0.,1.,0.));
#29460=DIRECTION('ref_axis',(1.,0.,0.));
#29461=DIRECTION('center_axis',(0.594611647405038,0.707106781186538,0.382670862191361));
#29462=DIRECTION('ref_axis',(0.541178323236022,-2.00621933738417E-16,-0.840907856105203));
#29463=DIRECTION('',(0.359954879607299,-0.659709210427941,0.659709210427926));
#29464=DIRECTION('',(0.541178323236022,0.,-0.840907856105203));
#29465=DIRECTION('',(-0.359954879607298,0.659709210427941,-0.659709210427927));
#29466=DIRECTION('center_axis',(0.,0.70710678118654,0.707106781186555));
#29467=DIRECTION('ref_axis',(1.,0.,0.));
#29468=DIRECTION('',(-0.577350269189623,-0.577350269189635,0.577350269189619));
#29469=DIRECTION('',(1.,0.,0.));
#29470=DIRECTION('center_axis',(-0.707106781186555,0.70710678118654,0.));
#29471=DIRECTION('ref_axis',(0.,0.,1.));
#29472=DIRECTION('',(-0.577350269189622,-0.577350269189635,-0.57735026918962));
#29473=DIRECTION('center_axis',(0.707106781186555,0.70710678118654,0.));
#29474=DIRECTION('ref_axis',(0.,0.,-1.));
#29475=DIRECTION('',(0.,0.,-1.));
#29476=DIRECTION('',(-0.577350269189622,0.577350269189634,-0.577350269189622));
#29477=DIRECTION('',(0.577350269189622,-0.577350269189634,-0.577350269189622));
#29478=DIRECTION('center_axis',(0.,0.70710678118654,-0.707106781186555));
#29479=DIRECTION('ref_axis',(-1.,0.,0.));
#29480=DIRECTION('',(-0.577350269189622,-0.577350269189634,-0.577350269189622));
#29481=DIRECTION('',(-1.,0.,0.));
#29482=DIRECTION('center_axis',(0.,0.70710678118654,0.707106781186555));
#29483=DIRECTION('ref_axis',(1.,0.,0.));
#29484=DIRECTION('',(-0.577350269189622,-0.577350269189635,0.57735026918962));
#29485=DIRECTION('',(1.,0.,0.));
#29486=DIRECTION('',(0.577350269189622,0.577350269189635,-0.57735026918962));
#29487=DIRECTION('center_axis',(-0.707106781186555,0.70710678118654,0.));
#29488=DIRECTION('ref_axis',(0.,0.,1.));
#29489=DIRECTION('',(-0.577350269189624,-0.577350269189633,-0.57735026918962));
#29490=DIRECTION('center_axis',(-0.594611647405038,0.707106781186538,-0.382670862191361));
#29491=DIRECTION('ref_axis',(-0.541178323236022,-2.00621933738417E-16,0.840907856105203));
#29492=DIRECTION('',(-0.541178323236022,0.,0.840907856105203));
#29493=DIRECTION('',(0.359954879607298,0.659709210427941,0.659709210427927));
#29494=DIRECTION('',(-0.359954879607299,-0.659709210427941,-0.659709210427926));
#29495=DIRECTION('center_axis',(0.,0.70710678118654,-0.707106781186555));
#29496=DIRECTION('ref_axis',(-1.,0.,0.));
#29497=DIRECTION('',(0.359954879607296,-0.659709210427942,-0.659709210427927));
#29498=DIRECTION('',(-1.,0.,0.));
#29499=DIRECTION('center_axis',(0.,0.70710678118654,-0.707106781186555));
#29500=DIRECTION('ref_axis',(-1.,0.,0.));
#29501=DIRECTION('',(-1.,0.,0.));
#29502=DIRECTION('',(-0.359954879607298,0.659709210427941,0.659709210427927));
#29503=DIRECTION('center_axis',(0.594611647405038,0.707106781186539,-0.382670862191361));
#29504=DIRECTION('ref_axis',(-0.541178323236022,1.9046781686272E-16,-0.840907856105203));
#29505=DIRECTION('',(-0.541178323236022,0.,-0.840907856105203));
#29506=DIRECTION('center_axis',(0.,0.70710678118654,-0.707106781186555));
#29507=DIRECTION('ref_axis',(-1.,0.,0.));
#29508=DIRECTION('',(-1.,0.,0.));
#29509=DIRECTION('',(0.577350269189623,-0.577350269189635,-0.577350269189619));
#29510=DIRECTION('center_axis',(0.707106781186555,0.70710678118654,0.));
#29511=DIRECTION('ref_axis',(0.,0.,-1.));
#29512=DIRECTION('',(0.577350269189622,-0.577350269189635,0.57735026918962));
#29513=DIRECTION('center_axis',(-0.707106781186555,0.70710678118654,0.));
#29514=DIRECTION('ref_axis',(0.,0.,1.));
#29515=DIRECTION('',(0.,0.,1.));
#29516=DIRECTION('center_axis',(0.,0.70710678118654,0.707106781186555));
#29517=DIRECTION('ref_axis',(1.,0.,0.));
#29518=DIRECTION('',(1.,0.,0.));
#29519=DIRECTION('center_axis',(0.,0.70710678118654,-0.707106781186555));
#29520=DIRECTION('ref_axis',(-1.,0.,0.));
#29521=DIRECTION('',(-1.,0.,0.));
#29522=DIRECTION('',(0.577350269189622,-0.577350269189635,-0.57735026918962));
#29523=DIRECTION('center_axis',(0.707106781186555,0.70710678118654,0.));
#29524=DIRECTION('ref_axis',(0.,0.,-1.));
#29525=DIRECTION('',(0.577350269189624,-0.577350269189633,0.57735026918962));
#29526=DIRECTION('center_axis',(0.,0.70710678118654,0.707106781186555));
#29527=DIRECTION('ref_axis',(1.,0.,0.));
#29528=DIRECTION('',(1.,0.,0.));
#29529=DIRECTION('',(-0.359954879607296,-0.659709210427942,0.659709210427927));
#29530=DIRECTION('center_axis',(0.,0.70710678118654,0.707106781186555));
#29531=DIRECTION('ref_axis',(1.,0.,0.));
#29532=DIRECTION('',(1.,0.,0.));
#29533=DIRECTION('',(0.359954879607298,0.659709210427941,-0.659709210427927));
#29534=DIRECTION('center_axis',(-0.594611647405038,0.707106781186539,0.382670862191361));
#29535=DIRECTION('ref_axis',(0.541178323236022,1.9046781686272E-16,0.840907856105203));
#29536=DIRECTION('',(0.541178323236022,0.,0.840907856105203));
#29537=DIRECTION('center_axis',(0.,0.,1.));
#29538=DIRECTION('ref_axis',(1.,0.,0.));
#29539=DIRECTION('',(-1.,0.,0.));
#29540=DIRECTION('',(0.,1.,0.));
#29541=DIRECTION('center_axis',(0.,0.,1.));
#29542=DIRECTION('ref_axis',(1.,0.,0.));
#29543=DIRECTION('',(0.,1.,0.));
#29544=DIRECTION('',(1.,0.,0.));
#29545=DIRECTION('center_axis',(1.,0.,0.));
#29546=DIRECTION('ref_axis',(0.,0.,-1.));
#29547=DIRECTION('',(0.,1.,0.));
#29548=DIRECTION('',(0.,0.,-1.));
#29549=DIRECTION('center_axis',(0.,0.,-1.));
#29550=DIRECTION('ref_axis',(-1.,0.,0.));
#29551=DIRECTION('',(-1.,0.,0.));
#29552=DIRECTION('center_axis',(0.,0.,-1.));
#29553=DIRECTION('ref_axis',(-1.,0.,0.));
#29554=DIRECTION('',(0.,-1.,0.));
#29555=DIRECTION('',(1.,0.,0.));
#29556=DIRECTION('center_axis',(-0.840907856105203,0.,0.541178323236022));
#29557=DIRECTION('ref_axis',(0.541178323236022,0.,0.840907856105203));
#29558=DIRECTION('',(0.,1.,0.));
#29559=DIRECTION('',(0.541178323236022,0.,0.840907856105203));
#29560=DIRECTION('center_axis',(0.,0.,1.));
#29561=DIRECTION('ref_axis',(1.,0.,0.));
#29562=DIRECTION('',(0.,1.,0.));
#29563=DIRECTION('',(1.,0.,0.));
#29564=DIRECTION('center_axis',(0.840907856105203,0.,0.541178323236022));
#29565=DIRECTION('ref_axis',(0.541178323236022,0.,-0.840907856105203));
#29566=DIRECTION('',(0.,1.,0.));
#29567=DIRECTION('',(0.541178323236022,0.,-0.840907856105203));
#29568=DIRECTION('center_axis',(0.840907856105203,0.,-0.541178323236022));
#29569=DIRECTION('ref_axis',(-0.541178323236022,0.,-0.840907856105203));
#29570=DIRECTION('',(0.,1.,0.));
#29571=DIRECTION('',(-0.541178323236022,0.,-0.840907856105203));
#29572=DIRECTION('',(0.,-1.,0.));
#29573=DIRECTION('center_axis',(-0.840907856105203,0.,-0.541178323236022));
#29574=DIRECTION('ref_axis',(-0.541178323236022,0.,0.840907856105203));
#29575=DIRECTION('',(-0.541178323236022,0.,0.840907856105203));
#29576=DIRECTION('',(0.,1.,0.));
#29577=DIRECTION('center_axis',(0.,0.,-1.));
#29578=DIRECTION('ref_axis',(-1.,0.,0.));
#29579=DIRECTION('',(-1.,0.,0.));
#29580=DIRECTION('center_axis',(0.,0.,-1.));
#29581=DIRECTION('ref_axis',(-1.,0.,0.));
#29582=DIRECTION('',(1.,0.,0.));
#29583=DIRECTION('center_axis',(0.,0.,1.));
#29584=DIRECTION('ref_axis',(1.,0.,0.));
#29585=DIRECTION('',(-1.,0.,0.));
#29586=DIRECTION('center_axis',(0.,1.,0.));
#29587=DIRECTION('ref_axis',(1.,0.,0.));
#29588=DIRECTION('',(-1.,0.,0.));
#29589=DIRECTION('',(0.,0.,1.));
#29590=DIRECTION('',(1.,0.,0.));
#29591=DIRECTION('center_axis',(-1.,0.,0.));
#29592=DIRECTION('ref_axis',(0.,0.,1.));
#29593=DIRECTION('',(0.,1.,0.));
#29594=DIRECTION('',(0.,1.,0.));
#29595=DIRECTION('center_axis',(0.,0.,-1.));
#29596=DIRECTION('ref_axis',(-1.,0.,0.));
#29597=DIRECTION('center_axis',(0.,0.,1.));
#29598=DIRECTION('ref_axis',(1.,0.,0.));
#36081=CARTESIAN_POINT('',(0.,0.,0.));
#36082=CARTESIAN_POINT('Origin',(-16.614,71.6454,-13.47));
#36083=CARTESIAN_POINT('',(-16.464,71.6454,-11.6675));
#36084=CARTESIAN_POINT('Origin',(-16.464,71.6454,-13.47));
#36085=CARTESIAN_POINT('',(-16.764,71.6454,-11.3675));
#36086=CARTESIAN_POINT('',(-16.614,71.6454,-11.5175));
#36087=CARTESIAN_POINT('Origin',(-16.764,71.6454,-13.47));
#36088=CARTESIAN_POINT('Origin',(-16.764,71.6454,-13.47));
#36089=CARTESIAN_POINT('',(-8.964,71.6454,-11.6675));
#36090=CARTESIAN_POINT('',(-16.764,71.6454,-11.6675));
#36091=CARTESIAN_POINT('',(-8.964,69.8429,-13.47));
#36092=CARTESIAN_POINT('Origin',(-8.964,71.6454,-13.47));
#36093=CARTESIAN_POINT('Origin',(-8.964,71.6454,-13.47));
#36094=CARTESIAN_POINT('Origin',(-16.764,68.4704,-16.51));
#36095=CARTESIAN_POINT('',(-16.764,74.4204,-16.51));
#36096=CARTESIAN_POINT('',(-16.764,74.4204,-8.13));
#36097=CARTESIAN_POINT('',(-16.764,74.4204,-8.255));
#36098=CARTESIAN_POINT('',(-16.764,68.4704,-16.51));
#36099=CARTESIAN_POINT('',(-16.764,68.4704,-16.51));
#36100=CARTESIAN_POINT('',(-16.764,68.4704,-8.13));
#36101=CARTESIAN_POINT('',(-16.764,68.4704,16.51));
#36102=CARTESIAN_POINT('',(-16.764,68.4704,-8.13));
#36103=CARTESIAN_POINT('Origin',(-16.614,71.6454,13.47));
#36104=CARTESIAN_POINT('',(-16.464,71.6454,15.2725));
#36105=CARTESIAN_POINT('Origin',(-16.464,71.6454,13.47));
#36106=CARTESIAN_POINT('',(-16.764,71.6454,15.5725));
#36107=CARTESIAN_POINT('',(-16.614,71.6454,15.4225));
#36108=CARTESIAN_POINT('Origin',(-16.764,71.6454,13.47));
#36109=CARTESIAN_POINT('Origin',(-16.764,71.6454,13.47));
#36110=CARTESIAN_POINT('',(-8.964,71.6454,15.2725));
#36111=CARTESIAN_POINT('',(-16.764,71.6454,15.2725));
#36112=CARTESIAN_POINT('',(-8.96400000000001,69.8429,13.47));
#36113=CARTESIAN_POINT('Origin',(-8.964,71.6454,13.47));
#36114=CARTESIAN_POINT('Origin',(-8.964,71.6454,13.47));
#36115=CARTESIAN_POINT('Origin',(-16.764,68.4704,-16.51));
#36116=CARTESIAN_POINT('',(-16.764,74.4204,8.13));
#36117=CARTESIAN_POINT('',(-16.764,74.4204,16.51));
#36118=CARTESIAN_POINT('',(-16.764,74.4204,-8.255));
#36119=CARTESIAN_POINT('',(-16.764,68.4704,8.13));
#36120=CARTESIAN_POINT('',(-16.764,68.4704,8.13));
#36121=CARTESIAN_POINT('',(-16.764,68.4704,16.51));
#36122=CARTESIAN_POINT('',(-16.764,68.4704,16.51));
#36123=CARTESIAN_POINT('',(-16.764,68.4704,16.51));
#36124=CARTESIAN_POINT('Origin',(-8.964,71.6454,-13.47));
#36125=CARTESIAN_POINT('',(-7.88094873420282,71.6454,-13.47));
#36126=CARTESIAN_POINT('',(-8.964,69.8429,-13.47));
#36127=CARTESIAN_POINT('Origin',(-8.964,71.6454,13.47));
#36128=CARTESIAN_POINT('',(-7.88094873420282,71.6454,13.47));
#36129=CARTESIAN_POINT('',(-8.964,69.8429,13.47));
#36130=CARTESIAN_POINT('Origin',(16.614,71.6454,-13.47));
#36131=CARTESIAN_POINT('',(16.464,71.6454,-11.6675));
#36132=CARTESIAN_POINT('Origin',(16.464,71.6454,-13.47));
#36133=CARTESIAN_POINT('',(16.764,71.6454,-11.3675));
#36134=CARTESIAN_POINT('',(16.614,71.6454,-11.5175));
#36135=CARTESIAN_POINT('Origin',(16.764,71.6454,-13.47));
#36136=CARTESIAN_POINT('Origin',(16.764,71.6454,-13.47));
#36137=CARTESIAN_POINT('',(8.964,71.6454,-11.6675));
#36138=CARTESIAN_POINT('',(16.764,71.6454,-11.6675));
#36139=CARTESIAN_POINT('',(8.964,69.8429,-13.47));
#36140=CARTESIAN_POINT('Origin',(8.964,71.6454,-13.47));
#36141=CARTESIAN_POINT('Origin',(8.964,71.6454,-13.47));
#36142=CARTESIAN_POINT('Origin',(16.764,68.4704,16.51));
#36143=CARTESIAN_POINT('',(16.764,74.4204,-8.13));
#36144=CARTESIAN_POINT('',(16.764,74.4204,-16.51));
#36145=CARTESIAN_POINT('',(16.764,74.4204,8.255));
#36146=CARTESIAN_POINT('',(16.764,68.4704,-8.13));
#36147=CARTESIAN_POINT('',(16.764,68.4704,-8.13));
#36148=CARTESIAN_POINT('',(16.764,68.4704,-16.51));
#36149=CARTESIAN_POINT('',(16.764,68.4704,-16.51));
#36150=CARTESIAN_POINT('',(16.764,68.4704,-16.51));
#36151=CARTESIAN_POINT('Origin',(16.614,71.6454,13.47));
#36152=CARTESIAN_POINT('',(16.464,71.6454,15.2725));
#36153=CARTESIAN_POINT('Origin',(16.464,71.6454,13.47));
#36154=CARTESIAN_POINT('',(16.764,71.6454,15.5725));
#36155=CARTESIAN_POINT('',(16.614,71.6454,15.4225));
#36156=CARTESIAN_POINT('Origin',(16.764,71.6454,13.47));
#36157=CARTESIAN_POINT('Origin',(16.764,71.6454,13.47));
#36158=CARTESIAN_POINT('',(8.964,71.6454,15.2725));
#36159=CARTESIAN_POINT('',(16.764,71.6454,15.2725));
#36160=CARTESIAN_POINT('',(8.964,69.8429,13.47));
#36161=CARTESIAN_POINT('Origin',(8.964,71.6454,13.47));
#36162=CARTESIAN_POINT('Origin',(8.964,71.6454,13.47));
#36163=CARTESIAN_POINT('Origin',(16.764,68.4704,16.51));
#36164=CARTESIAN_POINT('',(16.764,74.4204,16.51));
#36165=CARTESIAN_POINT('',(16.764,74.4204,8.13));
#36166=CARTESIAN_POINT('',(16.764,74.4204,8.255));
#36167=CARTESIAN_POINT('',(16.764,68.4704,16.51));
#36168=CARTESIAN_POINT('',(16.764,68.4704,16.51));
#36169=CARTESIAN_POINT('',(16.764,68.4704,8.13));
#36170=CARTESIAN_POINT('',(16.764,68.4704,-16.51));
#36171=CARTESIAN_POINT('',(16.764,68.4704,8.13));
#36172=CARTESIAN_POINT('Origin',(8.42247436710141,71.6454,-13.47));
#36173=CARTESIAN_POINT('',(7.88094873420282,71.6454,-13.47));
#36174=CARTESIAN_POINT('',(8.42247436710141,70.74415,-13.47));
#36175=CARTESIAN_POINT('Origin',(8.42247436710141,71.6454,13.47));
#36176=CARTESIAN_POINT('',(7.88094873420282,71.6454,13.47));
#36177=CARTESIAN_POINT('',(8.42247436710141,70.74415,13.47));
#36178=CARTESIAN_POINT('Origin',(6.91,74.8204,-6.91));
#36179=CARTESIAN_POINT('',(5.132,74.8204,-6.91));
#36180=CARTESIAN_POINT('Origin',(6.91,74.8204,-6.91));
#36181=CARTESIAN_POINT('',(5.132,68.4704,-6.91));
#36182=CARTESIAN_POINT('',(5.132,74.8204,-6.91));
#36183=CARTESIAN_POINT('Origin',(6.91,68.4704,-6.91));
#36184=CARTESIAN_POINT('Origin',(-6.91,74.8204,6.91));
#36185=CARTESIAN_POINT('',(-8.688,74.8204,6.91));
#36186=CARTESIAN_POINT('Origin',(-6.91,74.8204,6.91));
#36187=CARTESIAN_POINT('',(-8.688,68.4704,6.91));
#36188=CARTESIAN_POINT('',(-8.688,74.8204,6.91));
#36189=CARTESIAN_POINT('Origin',(-6.91,68.4704,6.91));
#36190=CARTESIAN_POINT('Origin',(6.91,74.8204,6.91));
#36191=CARTESIAN_POINT('',(5.132,74.8204,6.91));
#36192=CARTESIAN_POINT('Origin',(6.91,74.8204,6.91));
#36193=CARTESIAN_POINT('',(5.132,68.4704,6.91));
#36194=CARTESIAN_POINT('',(5.132,74.8204,6.91));
#36195=CARTESIAN_POINT('Origin',(6.91,68.4704,6.91));
#36196=CARTESIAN_POINT('Origin',(-6.91,74.8204,-6.91));
#36197=CARTESIAN_POINT('',(-8.688,74.8204,-6.91));
#36198=CARTESIAN_POINT('Origin',(-6.91,74.8204,-6.91));
#36199=CARTESIAN_POINT('',(-8.688,68.4704,-6.91));
#36200=CARTESIAN_POINT('',(-8.688,74.8204,-6.91));
#36201=CARTESIAN_POINT('Origin',(-6.91,68.4704,-6.91));
#36202=CARTESIAN_POINT('Origin',(-9.78,74.6704,0.));
#36203=CARTESIAN_POINT('',(-11.5825,74.5204,-2.2074258554631E-16));
#36204=CARTESIAN_POINT('Origin',(-9.78,74.5204,0.));
#36205=CARTESIAN_POINT('',(-11.8825,74.8204,2.57481989520731E-16));
#36206=CARTESIAN_POINT('',(-11.7325,74.6704,2.39112287533521E-16));
#36207=CARTESIAN_POINT('Origin',(-9.78,74.8204,0.));
#36208=CARTESIAN_POINT('Origin',(0.,74.8204,0.));
#36209=CARTESIAN_POINT('',(6.61825063159195,74.8204,-13.57));
#36210=CARTESIAN_POINT('',(8.25290409693848,74.8204,-16.11));
#36211=CARTESIAN_POINT('',(2.62042490592468,74.8204,-7.35799387242471));
#36212=CARTESIAN_POINT('',(-6.61825063159195,74.8204,-13.57));
#36213=CARTESIAN_POINT('',(-3.2,74.8204,-13.57));
#36214=CARTESIAN_POINT('',(-8.25290409693848,74.8204,-16.11));
#36215=CARTESIAN_POINT('',(-3.59542490592468,74.8204,-8.87299387242471));
#36216=CARTESIAN_POINT('',(-16.364,74.8204,-16.11));
#36217=CARTESIAN_POINT('',(8.382,74.8204,-16.11));
#36218=CARTESIAN_POINT('',(-16.364,74.8204,-8.53));
#36219=CARTESIAN_POINT('',(-16.364,74.8204,-8.255));
#36220=CARTESIAN_POINT('',(-13.07,74.8204,-8.53));
#36221=CARTESIAN_POINT('',(-6.735,74.8204,-8.53));
#36222=CARTESIAN_POINT('',(-13.07,74.8204,8.53));
#36223=CARTESIAN_POINT('',(-13.07,74.8204,4.065));
#36224=CARTESIAN_POINT('',(-16.364,74.8204,8.53));
#36225=CARTESIAN_POINT('',(-9.,74.8204,8.53));
#36226=CARTESIAN_POINT('',(-16.364,74.8204,16.11));
#36227=CARTESIAN_POINT('',(-16.364,74.8204,-8.255));
#36228=CARTESIAN_POINT('',(-8.25290409693848,74.8204,16.11));
#36229=CARTESIAN_POINT('',(-8.382,74.8204,16.11));
#36230=CARTESIAN_POINT('',(-6.61825063159195,74.8204,13.57));
#36231=CARTESIAN_POINT('',(-2.62042490592468,74.8204,7.35799387242471));
#36232=CARTESIAN_POINT('',(6.61825063159195,74.8204,13.57));
#36233=CARTESIAN_POINT('',(3.2,74.8204,13.57));
#36234=CARTESIAN_POINT('',(8.25290409693848,74.8204,16.11));
#36235=CARTESIAN_POINT('',(3.59542490592468,74.8204,8.87299387242471));
#36236=CARTESIAN_POINT('',(16.364,74.8204,16.11));
#36237=CARTESIAN_POINT('',(-8.382,74.8204,16.11));
#36238=CARTESIAN_POINT('',(16.364,74.8204,8.53));
#36239=CARTESIAN_POINT('',(16.364,74.8204,8.255));
#36240=CARTESIAN_POINT('',(13.07,74.8204,8.53));
#36241=CARTESIAN_POINT('',(6.735,74.8204,8.53));
#36242=CARTESIAN_POINT('',(13.07,74.8204,-8.53));
#36243=CARTESIAN_POINT('',(13.07,74.8204,-4.065));
#36244=CARTESIAN_POINT('',(16.364,74.8204,-8.53));
#36245=CARTESIAN_POINT('',(9.,74.8204,-8.53));
#36246=CARTESIAN_POINT('',(16.364,74.8204,-16.11));
#36247=CARTESIAN_POINT('',(16.364,74.8204,8.255));
#36248=CARTESIAN_POINT('',(8.382,74.8204,-16.11));
#36249=CARTESIAN_POINT('',(-2.1025,74.8204,-9.78));
#36250=CARTESIAN_POINT('Origin',(0.,74.8204,-9.78));
#36251=CARTESIAN_POINT('',(-6.763,74.8204,8.28228630263355E-16));
#36252=CARTESIAN_POINT('Origin',(0.,74.8204,0.));
#36253=CARTESIAN_POINT('',(7.6775,74.8204,2.57481989520731E-16));
#36254=CARTESIAN_POINT('Origin',(9.78,74.8204,0.));
#36255=CARTESIAN_POINT('',(-2.1025,74.8204,9.78));
#36256=CARTESIAN_POINT('Origin',(0.,74.8204,9.78));
#36257=CARTESIAN_POINT('Origin',(-9.78,74.8204,0.));
#36258=CARTESIAN_POINT('',(-11.5825,68.4704,2.2074258554631E-16));
#36259=CARTESIAN_POINT('',(-11.5825,74.8204,-2.2074258554631E-16));
#36260=CARTESIAN_POINT('Origin',(-9.78,68.4704,0.));
#36261=CARTESIAN_POINT('Origin',(0.,74.6704,9.78));
#36262=CARTESIAN_POINT('',(-1.8025,74.5204,9.78));
#36263=CARTESIAN_POINT('Origin',(0.,74.5204,9.78));
#36264=CARTESIAN_POINT('',(-1.9525,74.6704,9.78));
#36265=CARTESIAN_POINT('Origin',(0.,74.8204,9.78));
#36266=CARTESIAN_POINT('',(-1.8025,68.4704,9.78));
#36267=CARTESIAN_POINT('',(-1.8025,74.8204,9.78));
#36268=CARTESIAN_POINT('Origin',(0.,68.4704,9.78));
#36269=CARTESIAN_POINT('Origin',(0.,74.6704,-9.78));
#36270=CARTESIAN_POINT('',(-1.8025,74.5204,-9.78));
#36271=CARTESIAN_POINT('Origin',(0.,74.5204,-9.78));
#36272=CARTESIAN_POINT('',(-1.9525,74.6704,-9.78));
#36273=CARTESIAN_POINT('Origin',(0.,74.8204,-9.78));
#36274=CARTESIAN_POINT('',(-1.8025,68.4704,-9.78));
#36275=CARTESIAN_POINT('',(-1.8025,74.8204,-9.78));
#36276=CARTESIAN_POINT('Origin',(0.,68.4704,-9.78));
#36277=CARTESIAN_POINT('Origin',(9.78,74.6704,0.));
#36278=CARTESIAN_POINT('',(7.9775,74.5204,-2.2074258554631E-16));
#36279=CARTESIAN_POINT('Origin',(9.78,74.5204,0.));
#36280=CARTESIAN_POINT('',(7.8275,74.6704,2.39112287533521E-16));
#36281=CARTESIAN_POINT('Origin',(9.78,74.8204,0.));
#36282=CARTESIAN_POINT('',(7.9775,68.4704,2.2074258554631E-16));
#36283=CARTESIAN_POINT('',(7.9775,74.8204,-2.2074258554631E-16));
#36284=CARTESIAN_POINT('Origin',(9.78,68.4704,0.));
#36285=CARTESIAN_POINT('Origin',(0.,74.6204,0.));
#36286=CARTESIAN_POINT('',(-6.363,74.4204,-7.79242758297461E-16));
#36287=CARTESIAN_POINT('Origin',(0.,74.4204,0.));
#36288=CARTESIAN_POINT('',(-6.563,74.6204,8.03735694280408E-16));
#36289=CARTESIAN_POINT('Origin',(0.,74.8204,0.));
#36290=CARTESIAN_POINT('',(-6.363,68.4704,7.79242758297461E-16));
#36291=CARTESIAN_POINT('',(-6.363,74.8204,-7.79242758297461E-16));
#36292=CARTESIAN_POINT('Origin',(0.,68.4704,0.));
#36293=CARTESIAN_POINT('Origin',(-2.45224333470364,74.6204,7.46622953707191));
#36294=CARTESIAN_POINT('',(-8.03465346534654,74.4204,16.51));
#36295=CARTESIAN_POINT('',(-8.25290409693848,74.8204,16.11));
#36296=CARTESIAN_POINT('',(-6.4,74.4204,13.97));
#36297=CARTESIAN_POINT('',(-2.2840617634826,74.4204,7.57446520171912));
#36298=CARTESIAN_POINT('',(-6.4,74.4204,13.97));
#36299=CARTESIAN_POINT('Origin',(-8.382,74.6204,16.31));
#36300=CARTESIAN_POINT('',(-16.364,74.8204,16.11));
#36301=CARTESIAN_POINT('',(-8.382,74.4204,16.51));
#36302=CARTESIAN_POINT('Origin',(-16.564,74.6204,-8.255));
#36303=CARTESIAN_POINT('',(-16.364,74.8204,8.53));
#36304=CARTESIAN_POINT('Origin',(13.27,74.6204,-4.065));
#36305=CARTESIAN_POINT('',(13.47,74.4204,8.13));
#36306=CARTESIAN_POINT('',(13.47,74.4204,-8.13));
#36307=CARTESIAN_POINT('',(13.47,74.4204,-4.065));
#36308=CARTESIAN_POINT('',(13.47,74.4204,-8.13));
#36309=CARTESIAN_POINT('',(13.07,74.8204,8.53));
#36310=CARTESIAN_POINT('Origin',(-9.,74.6204,8.33));
#36311=CARTESIAN_POINT('',(-13.47,74.4204,8.13));
#36312=CARTESIAN_POINT('',(-13.07,74.8204,8.53));
#36313=CARTESIAN_POINT('',(-9.,74.4204,8.13));
#36314=CARTESIAN_POINT('Origin',(-6.735,74.6204,-8.33));
#36315=CARTESIAN_POINT('',(-16.364,74.8204,-8.53));
#36316=CARTESIAN_POINT('',(-13.47,74.4204,-8.13));
#36317=CARTESIAN_POINT('',(-6.735,74.4204,-8.13));
#36318=CARTESIAN_POINT('',(-13.47,74.4204,-8.13));
#36319=CARTESIAN_POINT('Origin',(-16.564,74.6204,-8.255));
#36320=CARTESIAN_POINT('',(-16.364,74.8204,-16.11));
#36321=CARTESIAN_POINT('Origin',(2.45224333470364,74.6204,-7.46622953707191));
#36322=CARTESIAN_POINT('',(8.03465346534654,74.4204,-16.51));
#36323=CARTESIAN_POINT('',(6.4,74.4204,-13.97));
#36324=CARTESIAN_POINT('',(2.2840617634826,74.4204,-7.57446520171912));
#36325=CARTESIAN_POINT('',(6.4,74.4204,-13.97));
#36326=CARTESIAN_POINT('',(8.25290409693848,74.8204,-16.11));
#36327=CARTESIAN_POINT('Origin',(8.382,74.6204,-16.31));
#36328=CARTESIAN_POINT('',(-8.03465346534654,74.4204,-16.51));
#36329=CARTESIAN_POINT('',(-8.25290409693848,74.8204,-16.11));
#36330=CARTESIAN_POINT('',(8.382,74.4204,-16.51));
#36331=CARTESIAN_POINT('Origin',(-3.2,74.6204,-13.77));
#36332=CARTESIAN_POINT('',(-6.4,74.4204,-13.97));
#36333=CARTESIAN_POINT('',(-3.2,74.4204,-13.97));
#36334=CARTESIAN_POINT('',(-6.4,74.4204,-13.97));
#36335=CARTESIAN_POINT('Origin',(-3.42724333470364,74.6204,-8.98122953707191));
#36336=CARTESIAN_POINT('',(-3.2590617634826,74.4204,-9.08946520171912));
#36337=CARTESIAN_POINT('Origin',(8.382,74.6204,-16.31));
#36338=CARTESIAN_POINT('',(8.382,74.4204,-16.51));
#36339=CARTESIAN_POINT('',(16.364,74.8204,-16.11));
#36340=CARTESIAN_POINT('Origin',(16.564,74.6204,8.255));
#36341=CARTESIAN_POINT('',(16.364,74.8204,-8.53));
#36342=CARTESIAN_POINT('Origin',(-13.27,74.6204,4.065));
#36343=CARTESIAN_POINT('',(-13.47,74.4204,4.065));
#36344=CARTESIAN_POINT('Origin',(9.,74.6204,-8.33));
#36345=CARTESIAN_POINT('',(9.,74.4204,-8.13));
#36346=CARTESIAN_POINT('Origin',(6.735,74.6204,8.33));
#36347=CARTESIAN_POINT('',(6.735,74.4204,8.13));
#36348=CARTESIAN_POINT('',(16.364,74.8204,8.53));
#36349=CARTESIAN_POINT('Origin',(16.564,74.6204,8.255));
#36350=CARTESIAN_POINT('',(16.364,74.8204,16.11));
#36351=CARTESIAN_POINT('Origin',(-8.382,74.6204,16.31));
#36352=CARTESIAN_POINT('',(8.03465346534654,74.4204,16.51));
#36353=CARTESIAN_POINT('',(-8.382,74.4204,16.51));
#36354=CARTESIAN_POINT('',(8.25290409693848,74.8204,16.11));
#36355=CARTESIAN_POINT('Origin',(3.2,74.6204,13.77));
#36356=CARTESIAN_POINT('',(6.4,74.4204,13.97));
#36357=CARTESIAN_POINT('',(3.2,74.4204,13.97));
#36358=CARTESIAN_POINT('',(6.4,74.4204,13.97));
#36359=CARTESIAN_POINT('Origin',(3.42724333470364,74.6204,8.98122953707191));
#36360=CARTESIAN_POINT('',(3.2590617634826,74.4204,9.08946520171912));
#36361=CARTESIAN_POINT('Origin',(-16.764,68.4704,16.51));
#36362=CARTESIAN_POINT('',(-8.03465346534653,68.4704,16.51));
#36363=CARTESIAN_POINT('',(16.764,68.4704,16.51));
#36364=CARTESIAN_POINT('',(-8.03465346534654,68.4704,16.51));
#36365=CARTESIAN_POINT('Origin',(-18.,68.4704,8.13));
#36366=CARTESIAN_POINT('',(-13.47,68.4704,8.13));
#36367=CARTESIAN_POINT('',(-13.47,68.4704,8.13));
#36368=CARTESIAN_POINT('',(-9.,68.4704,8.13));
#36369=CARTESIAN_POINT('Origin',(-13.47,68.4704,8.13));
#36370=CARTESIAN_POINT('',(-13.47,68.4704,-8.13));
#36371=CARTESIAN_POINT('',(-13.47,68.4704,-8.13));
#36372=CARTESIAN_POINT('',(-13.47,68.4704,4.065));
#36373=CARTESIAN_POINT('Origin',(-13.47,68.4704,-8.13));
#36374=CARTESIAN_POINT('',(-6.735,68.4704,-8.13));
#36375=CARTESIAN_POINT('Origin',(16.764,68.4704,-16.51));
#36376=CARTESIAN_POINT('',(-8.03465346534654,68.4704,-16.51));
#36377=CARTESIAN_POINT('',(-8.03465346534654,68.4704,-16.51));
#36378=CARTESIAN_POINT('',(-16.764,68.4704,-16.51));
#36379=CARTESIAN_POINT('Origin',(-8.35,68.4704,-17.));
#36380=CARTESIAN_POINT('',(-6.4,68.4704,-13.97));
#36381=CARTESIAN_POINT('',(-6.4,68.4704,-13.97));
#36382=CARTESIAN_POINT('',(-3.2590617634826,68.4704,-9.08946520171912));
#36383=CARTESIAN_POINT('Origin',(-6.4,68.4704,-13.97));
#36384=CARTESIAN_POINT('',(6.4,68.4704,-13.97));
#36385=CARTESIAN_POINT('',(6.4,68.4704,-13.97));
#36386=CARTESIAN_POINT('',(-3.2,68.4704,-13.97));
#36387=CARTESIAN_POINT('Origin',(6.4,68.4704,-13.97));
#36388=CARTESIAN_POINT('',(8.03465346534653,68.4704,-16.51));
#36389=CARTESIAN_POINT('',(8.03465346534654,68.4704,-16.51));
#36390=CARTESIAN_POINT('',(2.2840617634826,68.4704,-7.57446520171912));
#36391=CARTESIAN_POINT('Origin',(8.35,68.4704,17.));
#36392=CARTESIAN_POINT('',(6.4,68.4704,13.97));
#36393=CARTESIAN_POINT('',(6.4,68.4704,13.97));
#36394=CARTESIAN_POINT('',(8.03465346534654,68.4704,16.51));
#36395=CARTESIAN_POINT('',(3.2590617634826,68.4704,9.08946520171912));
#36396=CARTESIAN_POINT('',(8.03465346534654,68.4704,16.51));
#36397=CARTESIAN_POINT('Origin',(-6.4,68.4704,13.97));
#36398=CARTESIAN_POINT('',(-6.4,68.4704,13.97));
#36399=CARTESIAN_POINT('',(-2.2840617634826,68.4704,7.57446520171912));
#36400=CARTESIAN_POINT('',(-6.4,68.4704,13.97));
#36401=CARTESIAN_POINT('Origin',(6.4,68.4704,13.97));
#36402=CARTESIAN_POINT('',(3.2,68.4704,13.97));
#36403=CARTESIAN_POINT('Origin',(16.764,68.4704,-16.51));
#36404=CARTESIAN_POINT('',(-16.764,68.4704,-16.51));
#36405=CARTESIAN_POINT('Origin',(-16.764,68.4704,16.51));
#36406=CARTESIAN_POINT('',(16.764,68.4704,16.51));
#36407=CARTESIAN_POINT('Origin',(0.,68.4704,0.));
#36408=CARTESIAN_POINT('',(13.47,68.4704,-8.13));
#36409=CARTESIAN_POINT('',(9.,68.4704,-8.13));
#36410=CARTESIAN_POINT('',(13.47,68.4704,8.13));
#36411=CARTESIAN_POINT('',(13.47,68.4704,-4.065));
#36412=CARTESIAN_POINT('',(6.735,68.4704,8.13));
#36413=CARTESIAN_POINT('Origin',(13.47,68.4704,-8.13));
#36414=CARTESIAN_POINT('',(13.47,68.4704,8.13));
#36415=CARTESIAN_POINT('',(13.47,68.4704,-8.13));
#36416=CARTESIAN_POINT('Origin',(18.,68.4704,-8.13));
#36417=CARTESIAN_POINT('Origin',(13.47,68.4704,8.13));
#83189=UNCERTAINTY_MEASURE_WITH_UNIT(LENGTH_MEASURE(0.01),#83220,
'DISTANCE_ACCURACY_VALUE',
'Maximum model space distance between geometric entities at asserted c
onnectivities');
#83203=UNCERTAINTY_MEASURE_WITH_UNIT(LENGTH_MEASURE(0.01),#83220,
'DISTANCE_ACCURACY_VALUE',
'Maximum model space distance between geometric entities at asserted c
onnectivities');
#83205=(
GEOMETRIC_REPRESENTATION_CONTEXT(3)
GLOBAL_UNCERTAINTY_ASSIGNED_CONTEXT((#83189))
GLOBAL_UNIT_ASSIGNED_CONTEXT((#83220,#83222,#83223))
REPRESENTATION_CONTEXT('','3D')
);
#83219=(
GEOMETRIC_REPRESENTATION_CONTEXT(3)
GLOBAL_UNCERTAINTY_ASSIGNED_CONTEXT((#83203))
GLOBAL_UNIT_ASSIGNED_CONTEXT((#83220,#83222,#83223))
REPRESENTATION_CONTEXT('','3D')
);
#83220=(
LENGTH_UNIT()
NAMED_UNIT(*)
SI_UNIT(.MILLI.,.METRE.)
);
#83222=(
NAMED_UNIT(*)
PLANE_ANGLE_UNIT()
SI_UNIT($,.RADIAN.)
);
#83223=(
NAMED_UNIT(*)
SI_UNIT($,.STERADIAN.)
SOLID_ANGLE_UNIT()
);
#83225=SHAPE_DEFINITION_REPRESENTATION(#83240,#83300);
#83240=PRODUCT_DEFINITION_SHAPE('',$,#83316);
#83300=SHAPE_REPRESENTATION('',(#27099),#83205);
#83314=PRODUCT_DEFINITION_CONTEXT('part definition',#83361,'design');
#83316=PRODUCT_DEFINITION('90 Degree Quad Hub Mount B',
'90 Degree Quad Hub Mount B',#83331,#83314);
#83331=PRODUCT_DEFINITION_FORMATION('',$,#83364);
#83361=APPLICATION_CONTEXT(
'Core Data for Automotive Mechanical Design Process');
#83362=PRODUCT_CONTEXT('part definition',#83361,'mechanical');
#83364=PRODUCT('90 Degree Quad Hub Mount B',
'90 Degree Quad Hub Mount B',$,(#83362));
#83379=PRESENTATION_STYLE_ASSIGNMENT((#83394));
#83394=SURFACE_STYLE_USAGE(.BOTH.,#83409);
#83409=SURFACE_SIDE_STYLE('',(#83424));
#83424=SURFACE_STYLE_FILL_AREA(#83439);
#83439=FILL_AREA_STYLE('Opaque(222,225,230)',(#83454));
#83454=FILL_AREA_STYLE_COLOUR('Opaque(222,225,230)',#83469);
#83469=COLOUR_RGB('Opaque(222,225,230)', 0.66274510, 0.83137255, 0.94901961);
ENDSEC;
END-ISO-10303-21;
